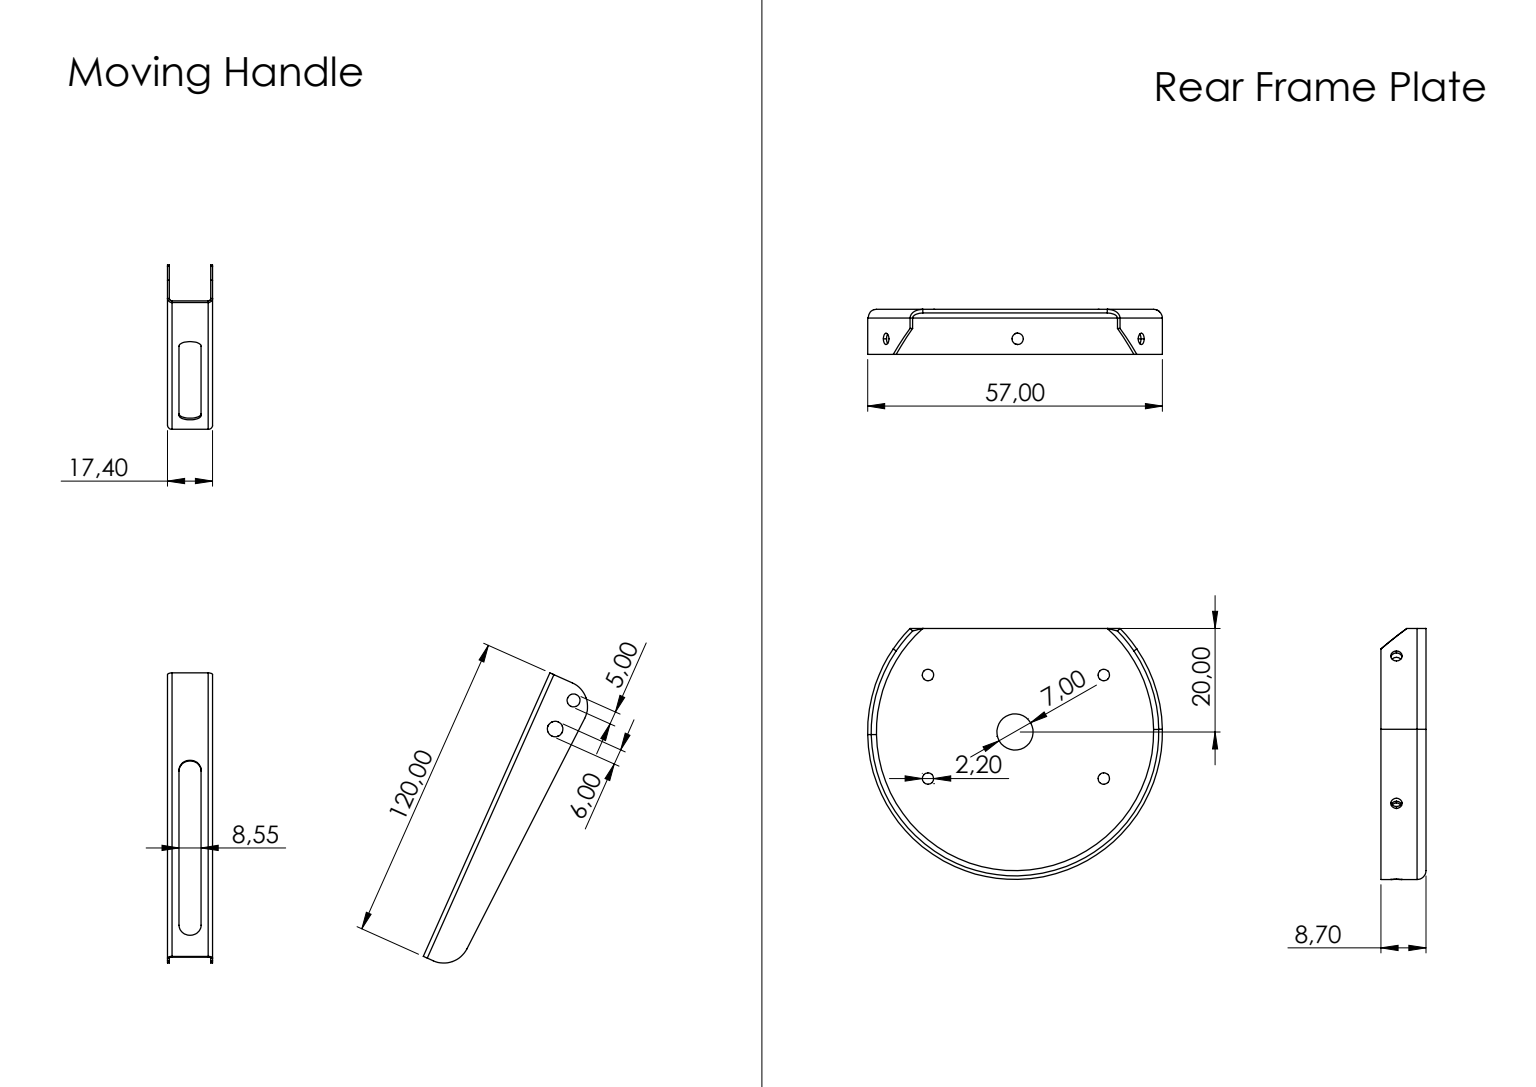
ISO-10303-21;
HEADER;
FILE_DESCRIPTION (('STEP AP214'),
    '1' );
FILE_NAME ('Moving Handle.step',
    '2026-10-06T09:00:30',
    ( '' ),
    ( '' ),
    'SwSTEP 2.0',
    'SolidWorks 2020',
    '' );
FILE_SCHEMA (( 'AUTOMOTIVE_DESIGN' ));
ENDSEC;

DATA;
#1=CARTESIAN_POINT ( 'NONE',  ( 7.707106781468556100, -5.692566302608600637, -27.29492475672613594 ) ) ;
#2=DIRECTION ( 'NONE',  ( 0.000000000000000000, 0.9128796883888953273, -0.4082287037029530552 ) ) ;
#16=VERTEX_POINT ( 'NONE', #10421 ) ;
#17=PRODUCT_DEFINITION ( 'UNKNOWN', '', #18877, #12195 ) ;
#34=DIRECTION ( 'NONE',  ( 1.000000000000000000, 3.839471067133294241E-11, -1.287095525146219562E-11 ) ) ;
#52=CARTESIAN_POINT ( 'NONE',  ( 1.057488903014505443E-10, -106.9648224075757952, 18.31364292107395642 ) ) ;
#61=VERTEX_POINT ( 'NONE', #24738 ) ;
#62=CARTESIAN_POINT ( 'NONE',  ( 7.707106781302665688, -60.46534760594231983, -2.801202534548945966 ) ) ;
#90=VERTEX_POINT ( 'NONE', #28021 ) ;
#95=DIRECTION ( 'NONE',  ( 2.764840495839172918E-12, 0.9128796883888953273, -0.4082287037029530552 ) ) ;
#99=CARTESIAN_POINT ( 'NONE',  ( 7.000000000111516130, -60.34578018690756807, -2.533826264242911908 ) ) ;
#105=DIRECTION ( 'NONE',  ( -1.000000000000000000, 5.687697937797165957E-16, -6.771501495045624776E-12 ) ) ;
#107=EDGE_CURVE ( 'NONE', #7680, #17625, #27535, .T. ) ;
#124=CARTESIAN_POINT ( 'NONE',  ( 7.291979204365766520, -115.1332600680515981, 21.92702704693240179 ) ) ;
#136=CARTESIAN_POINT ( 'NONE',  ( -7.000000000050451199, -115.5267901941139144, 21.04701626956108029 ) ) ;
#173=ORIENTED_EDGE ( 'NONE', *, *, #3047, .T. ) ;
#188=LINE ( 'NONE', #19684, #28372 ) ;
#203=ORIENTED_EDGE ( 'NONE', *, *, #5628, .T. ) ;
#223=DIRECTION ( 'NONE',  ( 1.000000000000000000, -1.843431230200084908E-12, 2.650498504963248473E-12 ) ) ;
#227=DIRECTION ( 'NONE',  ( 1.000000000000000000, -1.843431230200084908E-12, 2.650498504963248473E-12 ) ) ;
#233=LINE ( 'NONE', #19574, #18492 ) ;
#236=CARTESIAN_POINT ( 'NONE',  ( -8.000000000474178918, -29.73863906514523947, -27.17531388891475075 ) ) ;
#256=DIRECTION ( 'NONE',  ( -2.764840495839172918E-12, -0.9128796883888953273, 0.4082287037029531107 ) ) ;
#259=CARTESIAN_POINT ( 'NONE',  ( 8.000000000495651520, -23.99023929168359714, -28.09088344023833983 ) ) ;
#268=CARTESIAN_POINT ( 'NONE',  ( 8.700000000289421109, -16.34566964816854195, -38.02266470773063389 ) ) ;
#273=CARTESIAN_POINT ( 'NONE',  ( -8.699999999730765765, -25.41515418226572365, -25.82241997913822473 ) ) ;
#299=ORIENTED_EDGE ( 'NONE', *, *, #13486, .T. ) ;
#331=B_SPLINE_CURVE_WITH_KNOTS ( 'NONE', 4,
 ( #20135, #6279, #8153, #24861, #17748 ),
 .UNSPECIFIED., .F., .F.,
 ( 5, 5 ),
 ( -0.9817477042469999748, 0.9817477042469999748 ),
 .UNSPECIFIED. ) ;
#337=DIRECTION ( 'NONE',  ( -1.000000000000000000, 5.687697913155423197E-16, -6.771501495041734442E-12 ) ) ;
#360=LINE ( 'NONE', #2855, #2718 ) ;
#368=VERTEX_POINT ( 'NONE', #1564 ) ;
#371=ADVANCED_FACE ( 'NONE', ( #30354 ), #16338, .F. ) ;
#383=LINE ( 'NONE', #6989, #23905 ) ;
#402=EDGE_CURVE ( 'NONE', #3946, #1905, #1953, .T. ) ;
#419=CARTESIAN_POINT ( 'NONE',  ( 8.700000000293144353, -9.427296937348389250, -35.64651715365807405 ) ) ;
#421=EDGE_CURVE ( 'NONE', #12111, #14873, #20589, .T. ) ;
#435=LINE ( 'NONE', #22127, #18791 ) ;
#436=CARTESIAN_POINT ( 'NONE',  ( -7.999999999681902452, -14.92844969907143771, -33.25053330396754347 ) ) ;
#438=MANIFOLD_SOLID_BREP ( 'Stock-MAS-156-1', #10548 ) ;
#440=CARTESIAN_POINT ( 'NONE',  ( 7.665314379936610578, -115.2210683807244038, 21.73067038611315382 ) ) ;
#445=DIRECTION ( 'NONE',  ( -3.924189347185962345E-12, 0.4082287037029531107, 0.9128796883888953273 ) ) ;
#450=AXIS2_PLACEMENT_3D ( 'NONE', #30643, #26222, #11742 ) ;
#464=DIRECTION ( 'NONE',  ( -1.667070188605962886E-12, 0.4082287037029531107, 0.9128796883888953273 ) ) ;
#465=VECTOR ( 'NONE', #12974, 1000.000000000000000 ) ;
#469=DIRECTION ( 'NONE',  ( 2.764840495839172918E-12, 0.9128796883888953273, -0.4082287037029531107 ) ) ;
#475=CARTESIAN_POINT ( 'NONE',  ( 8.699999999949442397, -116.5561065468441626, 18.74526241745003574 ) ) ;
#492=DIRECTION ( 'NONE',  ( 6.325958275728752229E-12, 0.3568421334038983650, -0.9341647027306021478 ) ) ;
#496=EDGE_CURVE ( 'NONE', #28185, #6097, #18826, .T. ) ;
#531=CARTESIAN_POINT ( 'NONE',  ( -7.999999999670753148, -18.01685129643773564, -34.09892490238275542 ) ) ;
#545=CARTESIAN_POINT ( 'NONE',  ( -8.699999999716542476, -29.98791884354844939, -27.92359244214648228 ) ) ;
#555=CARTESIAN_POINT ( 'NONE',  ( -8.699999999672870743, -17.90468864316765973, -33.94136269864641520 ) ) ;
#575=CARTESIAN_POINT ( 'NONE',  ( -7.999999999684056284, -16.63651352361650382, -33.12749869627004529 ) ) ;
#597=ORIENTED_EDGE ( 'NONE', *, *, #20203, .T. ) ;
#605=VECTOR ( 'NONE', #18518, 1000.000000000000000 ) ;
#611=EDGE_LOOP ( 'NONE', ( #22896, #7545, #4645, #11032, #905, #16835, #7239, #10300 ) ) ;
#615=ADVANCED_FACE ( 'NONE', ( #10188, #8422, #29835 ), #7814, .F. ) ;
#617=CARTESIAN_POINT ( 'NONE',  ( 8.349999999579441834, -116.5561065468438215, 18.74526241744838373 ) ) ;
#624=CARTESIAN_POINT ( 'NONE',  ( -7.999999999945726081, -112.1477080532550445, 5.846459785100098117 ) ) ;
#657=CARTESIAN_POINT ( 'NONE',  ( 8.000000000883357387, -67.40749995174687115, -17.04319545456667484 ) ) ;
#713=EDGE_CURVE ( 'NONE', #20972, #5752, #15843, .T. ) ;
#714=CARTESIAN_POINT ( 'NONE',  ( -8.000000000001699973, -117.5009442568067755, 14.55791348096084192 ) ) ;
#725=VERTEX_POINT ( 'NONE', #10962 ) ;
#730=CARTESIAN_POINT ( 'NONE',  ( 7.000000000276031642, -5.430118837459354530, -26.70804059584096635 ) ) ;
#739=CARTESIAN_POINT ( 'NONE',  ( -7.999999999681398855, -14.76903124974032977, -33.32608274503188994 ) ) ;
#744=CYLINDRICAL_SURFACE ( 'NONE', #29818, 3.000000000000002220 ) ;
#754=CARTESIAN_POINT ( 'NONE',  ( -7.999999999888485647, -60.34578018689373380, -2.533826264313577603 ) ) ;
#757=CARTESIAN_POINT ( 'NONE',  ( 8.700000000279958456, -18.28438020625039329, -36.42481760783426381 ) ) ;
#773=CARTESIAN_POINT ( 'NONE',  ( -7.999999999947260854, -112.5823803020635125, 6.087179798330493163 ) ) ;
#775=DIRECTION ( 'NONE',  ( -1.000000000000000000, 5.687697999151106851E-16, -6.771501495036750356E-12 ) ) ;
#785=ORIENTED_EDGE ( 'NONE', *, *, #9500, .F. ) ;
#812=CARTESIAN_POINT ( 'NONE',  ( -8.699999999655181782, -13.66682223737418944, -36.55330428419230060 ) ) ;
#820=CARTESIAN_POINT ( 'NONE',  ( 7.785475348737113777, -115.2733928504967764, 21.61366257841296701 ) ) ;
#824=ORIENTED_EDGE ( 'NONE', *, *, #27429, .T. ) ;
#829=DIRECTION ( 'NONE',  ( 6.181308505765962611E-12, -0.4082287037029531107, -0.9128796883888953273 ) ) ;
#831=ORIENTED_EDGE ( 'NONE', *, *, #20654, .T. ) ;
#835=CARTESIAN_POINT ( 'NONE',  ( -7.999999999655180716, -13.66682223735657864, -36.55330428419717492 ) ) ;
#857=ORIENTED_EDGE ( 'NONE', *, *, #6995, .T. ) ;
#896=B_SPLINE_CURVE_WITH_KNOTS ( 'NONE', 3,
 ( #3635, #22846, #20952, #8825, #16225, #8506 ),
 .UNSPECIFIED., .F., .F.,
 ( 4, 2, 4 ),
 ( 0.000000000000000000, 0.5000000000000000000, 1.000000000000000000 ),
 .UNSPECIFIED. ) ;
#905=ORIENTED_EDGE ( 'NONE', *, *, #2120, .T. ) ;
#912=CARTESIAN_POINT ( 'NONE',  ( 8.700000000283074186, -17.54022835462044227, -37.48857263400110895 ) ) ;
#914=CYLINDRICAL_SURFACE ( 'NONE', #15454, 3.000000000000002220 ) ;
#945=CARTESIAN_POINT ( 'NONE',  ( 8.000000000289732682, -15.05691661385925961, -37.86814300156539304 ) ) ;
#950=DIRECTION ( 'NONE',  ( 3.924189347185962345E-12, -0.4082287037029530552, -0.9128796883888953273 ) ) ;
#954=DIRECTION ( 'NONE',  ( -1.000000000000000000, 5.687697999151106851E-16, -6.771501495036750356E-12 ) ) ;
#972=CARTESIAN_POINT ( 'NONE',  ( -7.999999999697742226, -24.65319937755806379, -30.30964379067835424 ) ) ;
#983=CARTESIAN_POINT ( 'NONE',  ( -7.999999999652784410, -17.12901166691730737, -37.73938230484767331 ) ) ;
#989=CARTESIAN_POINT ( 'NONE',  ( -7.999999999658122363, -13.45788390610263541, -35.88763790175109136 ) ) ;
#1016=EDGE_CURVE ( 'NONE', #725, #3834, #25246, .T. ) ;
#1017=CARTESIAN_POINT ( 'NONE',  ( -8.699999999945166707, -111.9817663798742444, 5.760339591697572814 ) ) ;
#1020=EDGE_CURVE ( 'NONE', #9868, #26249, #30013, .T. ) ;
#1081=DIRECTION ( 'NONE',  ( -1.000000000000000000, 5.687697999151106851E-16, -6.771501495036750356E-12 ) ) ;
#1113=EDGE_CURVE ( 'NONE', #7730, #30387, #4258, .T. ) ;
#1116=EDGE_LOOP ( 'NONE', ( #4416, #12493, #12956, #27444 ) ) ;
#1192=DIRECTION ( 'NONE',  ( 1.000000000000000000, -9.219999999999999084E-13, 4.710999999999999616E-12 ) ) ;
#1197=B_SPLINE_CURVE_WITH_KNOTS ( 'NONE', 3,
 ( #19881, #13084, #10731, #4703, #11053, #9258 ),
 .UNSPECIFIED., .F., .F.,
 ( 4, 2, 4 ),
 ( 0.000000000000000000, 0.5000000000000000000, 1.000000000000000000 ),
 .UNSPECIFIED. ) ;
#1198=EDGE_CURVE ( 'NONE', #2707, #23086, #13529, .T. ) ;
#1223=DIRECTION ( 'NONE',  ( 1.520059509754405802E-12, -0.4554456718803465698, -0.8902635789278700029 ) ) ;
#1253=FACE_OUTER_BOUND ( 'NONE', #18893, .T. ) ;
#1280=ORIENTED_EDGE ( 'NONE', *, *, #3659, .F. ) ;
#1289=DIRECTION ( 'NONE',  ( 1.000000000000000000, -1.843431230200084908E-12, 2.650498504963248473E-12 ) ) ;
#1311=DIRECTION ( 'NONE',  ( -1.000000000000000000, 5.687698019341907056E-16, -6.771501495046482653E-12 ) ) ;
#1331=CARTESIAN_POINT ( 'NONE',  ( 8.699999999994835420, -111.9817663798902885, 5.760339591779549018 ) ) ;
#1361=ORIENTED_EDGE ( 'NONE', *, *, #16817, .F. ) ;
#1401=ORIENTED_EDGE ( 'NONE', *, *, #2120, .F. ) ;
#1404=ADVANCED_FACE ( 'NONE', ( #13306 ), #27776, .F. ) ;
#1432=EDGE_LOOP ( 'NONE', ( #299, #9426, #4454, #14051 ) ) ;
#1440=CIRCLE ( 'NONE', #9974, 10.00000000000000355 ) ;
#1443=EDGE_CURVE ( 'NONE', #12111, #5252, #1887, .T. ) ;
#1446=CARTESIAN_POINT ( 'NONE',  ( -8.699999998997657968, -25.77531388886905006, -25.66136093486021608 ) ) ;
#1456=EDGE_LOOP ( 'NONE', ( #28511, #8580, #30468, #16902, #27099, #12265, #27129, #24342 ) ) ;
#1477=AXIS2_PLACEMENT_3D ( 'NONE', #30131, #20218, #29810 ) ;
#1480=DIRECTION ( 'NONE',  ( 3.134067079931429195E-12, 0.3568421334038983650, -0.9341647027306021478 ) ) ;
#1481=ORIENTED_EDGE ( 'NONE', *, *, #24442, .T. ) ;
#1509=CYLINDRICAL_SURFACE ( 'NONE', #21807, 2.500000000000000888 ) ;
#1512=DIRECTION ( 'NONE',  ( -3.924189347185963153E-12, 0.4082287037029530552, 0.9128796883888953273 ) ) ;
#1530=CARTESIAN_POINT ( 'NONE',  ( 8.000000000281330514, -5.981227587277713198, -27.94042817480428198 ) ) ;
#1538=CARTESIAN_POINT ( 'NONE',  ( -8.699999999715409160, -23.99014701217026513, -28.09041065100222312 ) ) ;
#1539=DIRECTION ( 'NONE',  ( -1.000000000000000000, 5.687697913153403713E-16, -6.771501495041734442E-12 ) ) ;
#1541=CARTESIAN_POINT ( 'NONE',  ( -7.999999999712662735, -24.01208138055985941, -28.87597782795289802 ) ) ;
#1542=PLANE ( 'NONE',  #10003 ) ;
#1546=CARTESIAN_POINT ( 'NONE',  ( 7.999999999977091214, -107.4273096626279482, 14.66297538114749344 ) ) ;
#1561=ORIENTED_EDGE ( 'NONE', *, *, #20981, .T. ) ;
#1562=EDGE_LOOP ( 'NONE', ( #10993, #30576, #17167, #18297 ) ) ;
#1564=CARTESIAN_POINT ( 'NONE',  ( -8.699999999681903518, -14.92844969908904851, -33.25053330396269047 ) ) ;
#1570=CARTESIAN_POINT ( 'NONE',  ( 8.000000000232340369, -25.77531388888444752, -25.66136093478154123 ) ) ;
#1575=ADVANCED_FACE ( 'NONE', ( #17176 ), #5217, .T. ) ;
#1599=CARTESIAN_POINT ( 'NONE',  ( -6.999999999262594308, -5.572998883415898774, -27.02754848611273530 ) ) ;
#1602=CARTESIAN_POINT ( 'NONE',  ( 8.000000000836740455, -15.37655846826601014, -33.05014450755139421 ) ) ;
#1617=LINE ( 'NONE', #20810, #27270 ) ;
#1628=ORIENTED_EDGE ( 'NONE', *, *, #2753, .F. ) ;
#1638=CARTESIAN_POINT ( 'NONE',  ( 8.699999999564820286, -13.66682223739023350, -36.55330428411032528 ) ) ;
#1646=CARTESIAN_POINT ( 'NONE',  ( 8.699999999979134202, -115.7892272573602668, 9.034522711534439310 ) ) ;
#1650=DIRECTION ( 'NONE',  ( -1.000000000000000000, 5.687697993419811493E-16, -6.771501495049272772E-12 ) ) ;
#1653=ORIENTED_EDGE ( 'NONE', *, *, #4274, .T. ) ;
#1675=ORIENTED_EDGE ( 'NONE', *, *, #19444, .T. ) ;
#1701=FACE_OUTER_BOUND ( 'NONE', #27105, .T. ) ;
#1705=ORIENTED_EDGE ( 'NONE', *, *, #20203, .F. ) ;
#1724=ORIENTED_EDGE ( 'NONE', *, *, #1020, .T. ) ;
#1729=B_SPLINE_CURVE_WITH_KNOTS ( 'NONE', 3,
 ( #3155, #17170, #5061, #26934, #19388, #7722 ),
 .UNSPECIFIED., .F., .F.,
 ( 4, 2, 4 ),
 ( 0.000000000000000000, 0.5000000000000000000, 1.000000000000000000 ),
 .UNSPECIFIED. ) ;
#1738=CARTESIAN_POINT ( 'NONE',  ( 7.614137047270383540, -5.654631194664418992, -27.21009439270542885 ) ) ;
#1748=VERTEX_POINT ( 'NONE', #6457 ) ;
#1754=ORIENTED_EDGE ( 'NONE', *, *, #30180, .F. ) ;
#1768=ORIENTED_EDGE ( 'NONE', *, *, #496, .F. ) ;
#1772=AXIS2_PLACEMENT_3D ( 'NONE', #11123, #11436, #18818 ) ;
#1787=DIRECTION ( 'NONE',  ( 1.000000000000000000, -9.219999999999999084E-13, 4.710999999999999616E-12 ) ) ;
#1789=ORIENTED_EDGE ( 'NONE', *, *, #16604, .F. ) ;
#1828=VERTEX_POINT ( 'NONE', #24929 ) ;
#1834=ORIENTED_EDGE ( 'NONE', *, *, #16604, .T. ) ;
#1842=CYLINDRICAL_SURFACE ( 'NONE', #13013, 2.500000000000002220 ) ;
#1869=CARTESIAN_POINT ( 'NONE',  ( 8.700000000277906764, -15.94902145836247342, -35.53273252485295330 ) ) ;
#1887=B_SPLINE_CURVE_WITH_KNOTS ( 'NONE', 3,
 ( #23076, #22606, #13141, #11110, #18341, #27943 ),
 .UNSPECIFIED., .F., .F.,
 ( 4, 2, 4 ),
 ( 0.000000000000000000, 0.5000000000000000000, 1.000000000000000000 ),
 .UNSPECIFIED. ) ;
#1891=CARTESIAN_POINT ( 'NONE',  ( 8.700000000233908182, -29.89969810940666406, -27.53547359536790395 ) ) ;
#1899=DIRECTION ( 'NONE',  ( -1.000000000000000000, 5.687697999151106851E-16, -6.771501495036750356E-12 ) ) ;
#1900=ORIENTED_EDGE ( 'NONE', *, *, #25212, .T. ) ;
#1903=EDGE_CURVE ( 'NONE', #19512, #21002, #23668, .T. ) ;
#1905=VERTEX_POINT ( 'NONE', #1017 ) ;
#1925=VECTOR ( 'NONE', #13869, 1000.000000000000000 ) ;
#1943=ORIENTED_EDGE ( 'NONE', *, *, #7815, .T. ) ;
#1953=B_SPLINE_CURVE_WITH_KNOTS ( 'NONE', 3,
 ( #25642, #6882, #11469, #4071, #21215, #11154 ),
 .UNSPECIFIED., .F., .F.,
 ( 4, 2, 4 ),
 ( 0.000000000000000000, 0.5000000000000001110, 1.000000000000000000 ),
 .UNSPECIFIED. ) ;
#1968=CARTESIAN_POINT ( 'NONE',  ( 8.000000000363138852, -29.66236253008535328, -29.83737202107615971 ) ) ;
#1978=ORIENTED_EDGE ( 'NONE', *, *, #2333, .F. ) ;
#2016=CARTESIAN_POINT ( 'NONE',  ( 8.700000000286559398, -7.565603753668719733, -31.48340496194444782 ) ) ;
#2049=CARTESIAN_POINT ( 'NONE',  ( -8.699999999715885224, -26.99999999997790923, -28.40000000002690683 ) ) ;
#2050=CYLINDRICAL_SURFACE ( 'NONE', #20849, 10.00000000000000178 ) ;
#2058=VERTEX_POINT ( 'NONE', #13425 ) ;
#2081=DIRECTION ( 'NONE',  ( 1.000000000000000000, -9.219999999999999084E-13, 4.710999999999999616E-12 ) ) ;
#2102=CARTESIAN_POINT ( 'NONE',  ( -8.699999999651183202, -14.46922738198402136, -37.57413277573995458 ) ) ;
#2105=AXIS2_PLACEMENT_3D ( 'NONE', #20895, #1223, #18035 ) ;
#2109=VECTOR ( 'NONE', #2270, 1000.000000000000114 ) ;
#2114=DIRECTION ( 'NONE',  ( 6.386904893851405129E-12, 0.3322662713817149949, -0.9431856258987901809 ) ) ;
#2120=EDGE_CURVE ( 'NONE', #17525, #17033, #24050, .T. ) ;
#2124=DIRECTION ( 'NONE',  ( 1.000000000000000000, -9.219999999999999084E-13, 4.710999999999999616E-12 ) ) ;
#2127=CARTESIAN_POINT ( 'NONE',  ( -7.999999999667107176, -18.39629690576770926, -34.94743992953217315 ) ) ;
#2150=UNCERTAINTY_MEASURE_WITH_UNIT (LENGTH_MEASURE( 1.000000000000000082E-05 ), #3991, 'distance_accuracy_value', 'NONE');
#2151=FACE_OUTER_BOUND ( 'NONE', #4462, .T. ) ;
#2152=EDGE_CURVE ( 'NONE', #27598, #22033, #3753, .T. ) ;
#2171=ORIENTED_EDGE ( 'NONE', *, *, #30137, .F. ) ;
#2178=B_SPLINE_CURVE_WITH_KNOTS ( 'NONE', 3,
 ( #4961, #2456, #259, #26825, #12502, #17072 ),
 .UNSPECIFIED., .F., .F.,
 ( 4, 2, 4 ),
 ( 0.000000000000000000, 0.5000000000000000000, 1.000000000000000000 ),
 .UNSPECIFIED. ) ;
#2182=AXIS2_PLACEMENT_3D ( 'NONE', #9189, #6836, #18789 ) ;
#2183=CARTESIAN_POINT ( 'NONE',  ( -8.699999999652812122, -10.55555246029782346, -37.33318641903195356 ) ) ;
#2184=CYLINDRICAL_SURFACE ( 'NONE', #12936, 2.500000000000000888 ) ;
#2214=CARTESIAN_POINT ( 'NONE',  ( -7.999999999655180716, -13.66682223735657864, -36.55330428419717492 ) ) ;
#2250=DIRECTION ( 'NONE',  ( 0.000000000000000000, -0.9128796883888953273, 0.4082287037029526666 ) ) ;
#2253=FACE_OUTER_BOUND ( 'NONE', #30967, .T. ) ;
#2259=ORIENTED_EDGE ( 'NONE', *, *, #7317, .T. ) ;
#2270=DIRECTION ( 'NONE',  ( -3.924189347185961537E-12, 0.4082287037029530552, 0.9128796883888952163 ) ) ;
#2280=B_SPLINE_CURVE_WITH_KNOTS ( 'NONE', 3,
 ( #9784, #15895, #15421, #20453, #18079, #8024 ),
 .UNSPECIFIED., .F., .F.,
 ( 4, 2, 4 ),
 ( 0.000000000000000000, 0.5000000000000000000, 1.000000000000000000 ),
 .UNSPECIFIED. ) ;
#2306=EDGE_LOOP ( 'NONE', ( #11495, #9641, #26655, #18802 ) ) ;
#2310=CARTESIAN_POINT ( 'NONE',  ( 8.700000000294076941, -9.763850040216345505, -36.23184806385972934 ) ) ;
#2333=EDGE_CURVE ( 'NONE', #23754, #8842, #22384, .T. ) ;
#2336=ORIENTED_EDGE ( 'NONE', *, *, #2412, .T. ) ;
#2357=CARTESIAN_POINT ( 'NONE',  ( 8.700000000235821318, -29.73863906516063693, -27.17531388883607590 ) ) ;
#2399=DIRECTION ( 'NONE',  ( -1.000000000000000000, 5.687697999151106851E-16, -6.771501495036750356E-12 ) ) ;
#2404=DIRECTION ( 'NONE',  ( 3.924189347185962345E-12, -0.4082287037029530552, -0.9128796883888953273 ) ) ;
#2412=EDGE_CURVE ( 'NONE', #16, #8184, #25150, .T. ) ;
#2420=FACE_OUTER_BOUND ( 'NONE', #9603, .T. ) ;
#2430=DIRECTION ( 'NONE',  ( -1.000000000000000000, 5.687697999151106851E-16, -6.771501495036750356E-12 ) ) ;
#2432=B_SPLINE_CURVE_WITH_KNOTS ( 'NONE', 3,
 ( #19714, #2564, #21611, #14683, #5225, #7127 ),
 .UNSPECIFIED., .F., .F.,
 ( 4, 2, 4 ),
 ( 0.000000000000000000, 0.5000000000000000000, 1.000000000000000000 ),
 .UNSPECIFIED. ) ;
#2445=ORIENTED_EDGE ( 'NONE', *, *, #24054, .T. ) ;
#2456=CARTESIAN_POINT ( 'NONE',  ( 8.000000000368686415, -24.05737431370143398, -27.69631922065391905 ) ) ;
#2459=CARTESIAN_POINT ( 'NONE',  ( 8.700000000285857737, -13.61366271048277277, -34.64064744186795508 ) ) ;
#2499=VERTEX_POINT ( 'NONE', #30665 ) ;
#2515=B_SPLINE_CURVE_WITH_KNOTS ( 'NONE', 3,
 ( #4871, #10058, #7677, #23925, #12407, #475 ),
 .UNSPECIFIED., .F., .F.,
 ( 4, 2, 4 ),
 ( 0.000000000000000000, 0.5000000000000000000, 1.000000000000000000 ),
 .UNSPECIFIED. ) ;
#2529=FACE_OUTER_BOUND ( 'NONE', #4143, .T. ) ;
#2532=CARTESIAN_POINT ( 'NONE',  ( -8.699999999662093586, -15.94902145834643115, -35.53273252493492862 ) ) ;
#2542=DIRECTION ( 'NONE',  ( 1.000000000000000000, -1.843431230200084908E-12, 2.650498504963248473E-12 ) ) ;
#2564=CARTESIAN_POINT ( 'NONE',  ( -7.799123028745747810, -5.730129976181659757, -27.37892452043196556 ) ) ;
#2567=CARTESIAN_POINT ( 'NONE',  ( -4.276011752185619130, -110.9401521130015027, -1.050525799534463012 ) ) ;
#2576=B_SPLINE_CURVE_WITH_KNOTS ( 'NONE', 3,
 ( #4173, #18790, #11253, #21474, #16438, #9190 ),
 .UNSPECIFIED., .F., .F.,
 ( 4, 2, 4 ),
 ( 0.000000000000000000, 0.5000000000000000000, 1.000000000000000000 ),
 .UNSPECIFIED. ) ;
#2605=CARTESIAN_POINT ( 'NONE',  ( -7.999999999682589014, -15.17486759261230311, -33.15315993661145910 ) ) ;
#2609=CARTESIAN_POINT ( 'NONE',  ( 8.700000000287717583, -16.96959321760160222, -37.81493174583334849 ) ) ;
#2615=CARTESIAN_POINT ( 'NONE',  ( -8.699999999718343702, -24.19750589173278499, -27.32947359979484858 ) ) ;
#2619=EDGE_CURVE ( 'NONE', #16921, #22622, #17600, .T. ) ;
#2627=CARTESIAN_POINT ( 'NONE',  ( 0.000000000000000000, 0.000000000000000000, 0.000000000000000000 ) ) ;
#2638=( NAMED_UNIT ( * ) SI_UNIT ( $, .STERADIAN. ) SOLID_ANGLE_UNIT ( ) );
#2641=DIRECTION ( 'NONE',  ( -1.000000000000000000, 5.687698019341907056E-16, -6.771501495046482653E-12 ) ) ;
#2651=VECTOR ( 'NONE', #7343, 1000.000000000000114 ) ;
#2669=ORIENTED_EDGE ( 'NONE', *, *, #30970, .T. ) ;
#2673=CARTESIAN_POINT ( 'NONE',  ( -7.999999999729513256, -26.54727805893419657, -25.41789611383235226 ) ) ;
#2689=EDGE_CURVE ( 'NONE', #18386, #18002, #22877, .T. ) ;
#2707=VERTEX_POINT ( 'NONE', #11920 ) ;
#2717=CARTESIAN_POINT ( 'NONE',  ( -7.999999999683915952, -16.84112630284391443, -33.19732204833458411 ) ) ;
#2718=VECTOR ( 'NONE', #4910, 1000.000000000000000 ) ;
#2753=EDGE_CURVE ( 'NONE', #15244, #5752, #12004, .T. ) ;
#2756=VERTEX_POINT ( 'NONE', #10496 ) ;
#2770=CYLINDRICAL_SURFACE ( 'NONE', #28345, 3.000000000000002220 ) ;
#2785=VERTEX_POINT ( 'NONE', #21181 ) ;
#2801=CARTESIAN_POINT ( 'NONE',  ( 8.700000000244115128, -26.99999999999395328, -28.39999999994493862 ) ) ;
#2821=ORIENTED_EDGE ( 'NONE', *, *, #9836, .F. ) ;
#2855=CARTESIAN_POINT ( 'NONE',  ( 8.699999999511655702, -24.19750589174882904, -27.32947359971288037 ) ) ;
#2866=CARTESIAN_POINT ( 'NONE',  ( 8.700000000252410715, -24.26136093482726608, -29.62468611105379779 ) ) ;
#2868=DIRECTION ( 'NONE',  ( -3.924189347185962345E-12, 0.4082287037029531107, 0.9128796883888953273 ) ) ;
#2879=LINE ( 'NONE', #28840, #12838 ) ;
#2908=EDGE_CURVE ( 'NONE', #13888, #17663, #7099, .T. ) ;
#2913=EDGE_CURVE ( 'NONE', #23040, #9577, #12648, .T. ) ;
#2914=CARTESIAN_POINT ( 'NONE',  ( -7.999999999668208517, -9.149979920084513552, -35.02638174925785819 ) ) ;
#2924=AXIS2_PLACEMENT_3D ( 'NONE', #17301, #337, #492 ) ;
#2957=VECTOR ( 'NONE', #27758, 999.9999999999998863 ) ;
#2967=ADVANCED_FACE ( 'NONE', ( #20992 ), #9023, .F. ) ;
#2969=LINE ( 'NONE', #15231, #26882 ) ;
#2989=CARTESIAN_POINT ( 'NONE',  ( 5.797918472256613498, -5.490503403373238278, -26.84307236410781172 ) ) ;
#2998=CARTESIAN_POINT ( 'NONE',  ( -6.999999999884560786, -60.75400889059761766, -3.446705952697758590 ) ) ;
#3021=CARTESIAN_POINT ( 'NONE',  ( -7.999999999659364924, -18.23057825131764531, -36.55854538514943641 ) ) ;
#3022=ORIENTED_EDGE ( 'NONE', *, *, #2152, .T. ) ;
#3036=CARTESIAN_POINT ( 'NONE',  ( -8.699999999786642846, -67.40749995144571471, -17.04319545400634084 ) ) ;
#3043=FACE_OUTER_BOUND ( 'NONE', #28369, .T. ) ;
#3047=EDGE_CURVE ( 'NONE', #3834, #17179, #12007, .T. ) ;
#3055=DIRECTION ( 'NONE',  ( 0.000000000000000000, -0.9128796883888952163, 0.4082287037029533328 ) ) ;
#3113=CYLINDRICAL_SURFACE ( 'NONE', #30869, 2.500000000000001776 ) ;
#3128=APPLICATION_CONTEXT ( 'automotive_design' ) ;
#3134=LINE ( 'NONE', #19975, #24510 ) ;
#3137=LINE ( 'NONE', #12736, #9564 ) ;
#3152=CARTESIAN_POINT ( 'NONE',  ( -8.699999999674142614, -13.61360970150653316, -34.64062719139432289 ) ) ;
#3155=CARTESIAN_POINT ( 'NONE',  ( 8.000000000232340369, -25.77531388888444752, -25.66136093478154123 ) ) ;
#3194=CARTESIAN_POINT ( 'NONE',  ( -8.699999999677118012, -17.14683147485207471, -33.31409708255895907 ) ) ;
#3207=CARTESIAN_POINT ( 'NONE',  ( -8.000000000018781421, -117.3918542544958115, 16.08262865818876008 ) ) ;
#3253=LINE ( 'NONE', #29532, #5771 ) ;
#3259=DIRECTION ( 'NONE',  ( -1.000000000000000000, 5.687698019341907056E-16, -6.771501495046482653E-12 ) ) ;
#3284=ADVANCED_FACE ( 'NONE', ( #12463 ), #24900, .F. ) ;
#3323=CARTESIAN_POINT ( 'NONE',  ( -7.999999999655324601, -17.72367216628370556, -37.31664291223312091 ) ) ;
#3337=B_SPLINE_CURVE_WITH_KNOTS ( 'NONE', 3,
 ( #14013, #16823, #11646, #26274, #23618, #4410 ),
 .UNSPECIFIED., .F., .F.,
 ( 4, 2, 4 ),
 ( 0.000000000000000000, 0.5000000000000000000, 1.000000000000000000 ),
 .UNSPECIFIED. ) ;
#3356=CARTESIAN_POINT ( 'NONE',  ( -7.999999999988746779, -117.0548398251480364, 11.89578701954164686 ) ) ;
#3369=ORIENTED_EDGE ( 'NONE', *, *, #14073, .T. ) ;
#3390=DIRECTION ( 'NONE',  ( 2.764840495839172918E-12, 0.9128796883888953273, -0.4082287037029531107 ) ) ;
#3399=EDGE_CURVE ( 'NONE', #29694, #1748, #3493, .T. ) ;
#3428=ADVANCED_FACE ( 'NONE', ( #21893 ), #21580, .F. ) ;
#3461=CARTESIAN_POINT ( 'NONE',  ( -7.999999999728557576, -25.41682687375232064, -25.82167197182654661 ) ) ;
#3471=AXIS2_PLACEMENT_3D ( 'NONE', #22262, #26521, #24015 ) ;
#3484=ORIENTED_EDGE ( 'NONE', *, *, #21630, .T. ) ;
#3493=B_SPLINE_CURVE_WITH_KNOTS ( 'NONE', 3,
 ( #6468, #14181, #18736, #17000, #14346, #12276 ),
 .UNSPECIFIED., .F., .F.,
 ( 4, 2, 4 ),
 ( 0.000000000000000000, 0.5000000000000000000, 1.000000000000000000 ),
 .UNSPECIFIED. ) ;
#3494=VECTOR ( 'NONE', #22040, 1000.000000000000114 ) ;
#3501=FACE_OUTER_BOUND ( 'NONE', #30433, .T. ) ;
#3528=CARTESIAN_POINT ( 'NONE',  ( 7.000000000108768994, -60.06002009431549737, -1.894810482370685278 ) ) ;
#3550=B_SPLINE_CURVE_WITH_KNOTS ( 'NONE', 5,
 ( #29442, #22375, #22215, #820, #14831, #10410, #17480, #17778, #27391, #5830, #21918, #19549 ),
 .UNSPECIFIED., .F., .F.,
 ( 6, 3, 3, 6 ),
 ( 1.117931991990000151, 1.394586747660000015, 2.091870620439999939, 2.235835859519999858 ),
 .UNSPECIFIED. ) ;
#3556=CARTESIAN_POINT ( 'NONE',  ( 8.700000000294906499, -15.59658250094199161, -40.60120179151234510 ) ) ;
#3562=CARTESIAN_POINT ( 'NONE',  ( -8.699999999715885224, -26.99999999997790923, -28.40000000002690683 ) ) ;
#3585=ORIENTED_EDGE ( 'NONE', *, *, #14607, .F. ) ;
#3586=EDGE_CURVE ( 'NONE', #30810, #24995, #3137, .T. ) ;
#3600=ORIENTED_EDGE ( 'NONE', *, *, #18462, .F. ) ;
#3606=LINE ( 'NONE', #29737, #24715 ) ;
#3621=ORIENTED_EDGE ( 'NONE', *, *, #7436, .T. ) ;
#3623=VERTEX_POINT ( 'NONE', #1570 ) ;
#3634=PLANE ( 'NONE',  #23108 ) ;
#3635=CARTESIAN_POINT ( 'NONE',  ( -8.699999999642283655, -16.96959321760381556, -37.81493174590716677 ) ) ;
#3651=VERTEX_POINT ( 'NONE', #30193 ) ;
#3654=CARTESIAN_POINT ( 'NONE',  ( -8.699999999662093586, -15.94902145834643115, -35.53273252493492862 ) ) ;
#3659=EDGE_CURVE ( 'NONE', #15429, #30761, #24134, .T. ) ;
#3666=VERTEX_POINT ( 'NONE', #18221 ) ;
#3685=LINE ( 'NONE', #8391, #465 ) ;
#3711=ORIENTED_EDGE ( 'NONE', *, *, #10079, .T. ) ;
#3714=VECTOR ( 'NONE', #13963, 1000.000000000000000 ) ;
#3730=CARTESIAN_POINT ( 'NONE',  ( -7.999999999710018628, -24.10104989765104833, -29.26619909559191157 ) ) ;
#3753=B_SPLINE_CURVE_WITH_KNOTS ( 'NONE', 3,
 ( #19400, #5074, #2102, #28378, #9329, #9639 ),
 .UNSPECIFIED., .F., .F.,
 ( 4, 2, 4 ),
 ( 0.000000000000000000, 0.5000000000000000000, 1.000000000000000000 ),
 .UNSPECIFIED. ) ;
#3776=CARTESIAN_POINT ( 'NONE',  ( -7.999999999627967817, -15.63018644032419857, -40.59129444282516630 ) ) ;
#3801=DIRECTION ( 'NONE',  ( 1.000000000000000000, -1.843431230200084908E-12, 2.650498504963248473E-12 ) ) ;
#3834=VERTEX_POINT ( 'NONE', #21075 ) ;
#3850=ORIENTED_EDGE ( 'NONE', *, *, #27186, .F. ) ;
#3861=CARTESIAN_POINT ( 'NONE',  ( 6.999999999814658480, -5.287238791122498505, -26.38853270481357072 ) ) ;
#3869=DIRECTION ( 'NONE',  ( -2.415891560877031462E-12, 0.9341647027306021478, 0.3568421334038983650 ) ) ;
#3884=EDGE_CURVE ( 'NONE', #9121, #31008, #331, .T. ) ;
#3890=CARTESIAN_POINT ( 'NONE',  ( -8.699999999662093586, -15.94902145834643115, -35.53273252493492862 ) ) ;
#3906=VERTEX_POINT ( 'NONE', #25005 ) ;
#3908=ORIENTED_EDGE ( 'NONE', *, *, #13956, .T. ) ;
#3938=CYLINDRICAL_SURFACE ( 'NONE', #14271, 3.000000000000002220 ) ;
#3942=ORIENTED_EDGE ( 'NONE', *, *, #2689, .F. ) ;
#3946=VERTEX_POINT ( 'NONE', #30192 ) ;
#3956=CARTESIAN_POINT ( 'NONE',  ( 8.000000000465679051, -16.38256976572606405, -33.02215629541608877 ) ) ;
#3967=ADVANCED_FACE ( 'NONE', ( #1253 ), #18220, .T. ) ;
#3968=CARTESIAN_POINT ( 'NONE',  ( 7.999999999944494178, -116.0414483704652042, 19.89613934358488123 ) ) ;
#3991=( LENGTH_UNIT ( ) NAMED_UNIT ( * ) SI_UNIT ( .MILLI., .METRE. ) );
#4003=AXIS2_PLACEMENT_3D ( 'NONE', #754, #10646, #20238 ) ;
#4015=CARTESIAN_POINT ( 'NONE',  ( 8.000000000270995670, -18.23122067931581114, -34.51216076560703527 ) ) ;
#4042=FACE_OUTER_BOUND ( 'NONE', #18444, .T. ) ;
#4048=EDGE_CURVE ( 'NONE', #22923, #2058, #13991, .T. ) ;
#4060=CARTESIAN_POINT ( 'NONE',  ( -8.699999999642283655, -16.96959321760381556, -37.81493174590716677 ) ) ;
#4071=CARTESIAN_POINT ( 'NONE',  ( -8.699999999957434227, -114.1237136948164306, 7.129097339259313770 ) ) ;
#4073=CARTESIAN_POINT ( 'NONE',  ( -8.699999999664235872, -9.427153351153990002, -35.64619606679892883 ) ) ;
#4096=FACE_OUTER_BOUND ( 'NONE', #20301, .T. ) ;
#4136=EDGE_LOOP ( 'NONE', ( #10645, #7084, #21287, #19421 ) ) ;
#4138=DIRECTION ( 'NONE',  ( -3.927995826131583318E-12, 0.4082287037029531107, 0.9128796883888953273 ) ) ;
#4140=VECTOR ( 'NONE', #22590, 1000.000000000000000 ) ;
#4143=EDGE_LOOP ( 'NONE', ( #17592, #28862, #14441, #6769 ) ) ;
#4168=CARTESIAN_POINT ( 'NONE',  ( -8.699999999681903518, -14.92844969908904851, -33.25053330396269047 ) ) ;
#4173=CARTESIAN_POINT ( 'NONE',  ( 8.000000000245886866, -28.22468611110216230, -31.13863906511491209 ) ) ;
#4202=FACE_OUTER_BOUND ( 'NONE', #28460, .T. ) ;
#4212=CARTESIAN_POINT ( 'NONE',  ( 8.699999999974050269, -116.8589940799748632, 11.34037320843244956 ) ) ;
#4237=VERTEX_POINT ( 'NONE', #29840 ) ;
#4243=CARTESIAN_POINT ( 'NONE',  ( 8.000000000480120832, -27.30911655970313845, -25.39023929163792204 ) ) ;
#4244=CARTESIAN_POINT ( 'NONE',  ( -6.999999999718670374, -5.981227587263883372, -27.94042817487494901 ) ) ;
#4249=EDGE_CURVE ( 'NONE', #24850, #24204, #4401, .T. ) ;
#4258=LINE ( 'NONE', #27857, #13061 ) ;
#4274=EDGE_CURVE ( 'NONE', #22839, #9868, #3253, .T. ) ;
#4287=CYLINDRICAL_SURFACE ( 'NONE', #12133, 1.700000000000000178 ) ;
#4301=B_SPLINE_CURVE_WITH_KNOTS ( 'NONE', 3,
 ( #27035, #10514, #12707, #20113, #19953, #5472 ),
 .UNSPECIFIED., .F., .F.,
 ( 4, 2, 4 ),
 ( 0.000000000000000000, 0.5000000000000000000, 1.000000000000000000 ),
 .UNSPECIFIED. ) ;
#4306=ORIENTED_EDGE ( 'NONE', *, *, #7347, .F. ) ;
#4314=DIRECTION ( 'NONE',  ( 6.325958275728752229E-12, 0.3568421334038983650, -0.9341647027306021478 ) ) ;
#4320=CYLINDRICAL_SURFACE ( 'NONE', #21877, 10.00000000000000533 ) ;
#4328=ADVANCED_FACE ( 'NONE', ( #2151 ), #23091, .F. ) ;
#4333=DIRECTION ( 'NONE',  ( -3.924189347185963153E-12, 0.4082287037029530552, 0.9128796883888953273 ) ) ;
#4355=DIRECTION ( 'NONE',  ( -1.000000000000000000, 5.687697913153403713E-16, -6.771501495041734442E-12 ) ) ;
#4358=PLANE ( 'NONE',  #6731 ) ;
#4367=DIRECTION ( 'NONE',  ( -1.667070188605962886E-12, 0.4082287037029531107, 0.9128796883888953273 ) ) ;
#4378=PRODUCT_DEFINITION_SHAPE ( 'NONE', 'NONE',  #17 ) ;
#4381=EDGE_CURVE ( 'NONE', #10063, #17033, #16761, .T. ) ;
#4382=FACE_OUTER_BOUND ( 'NONE', #11513, .T. ) ;
#4397=CARTESIAN_POINT ( 'NONE',  ( -7.999999999629061165, -18.86445920977251234, -40.99220581062246538 ) ) ;
#4401=B_SPLINE_CURVE_WITH_KNOTS ( 'NONE', 3,
 ( #17712, #15214, #912, #27331, #5769, #757 ),
 .UNSPECIFIED., .F., .F.,
 ( 4, 2, 4 ),
 ( 0.000000000000000000, 0.5000000000000000000, 1.000000000000000000 ),
 .UNSPECIFIED. ) ;
#4405=EDGE_CURVE ( 'NONE', #6605, #27863, #11543, .T. ) ;
#4410=CARTESIAN_POINT ( 'NONE',  ( 8.700000000252410715, -24.26136093482726608, -29.62468611105379779 ) ) ;
#4416=ORIENTED_EDGE ( 'NONE', *, *, #14650, .T. ) ;
#4423=EDGE_CURVE ( 'NONE', #1748, #23469, #28453, .T. ) ;
#4442=ADVANCED_FACE ( 'NONE', ( #28884 ), #24316, .T. ) ;
#4452=CARTESIAN_POINT ( 'NONE',  ( 8.700000000241654874, -24.19757157926353486, -27.32949869323976699 ) ) ;
#4454=ORIENTED_EDGE ( 'NONE', *, *, #13252, .F. ) ;
#4458=VERTEX_POINT ( 'NONE', #2914 ) ;
#4460=SURFACE_SIDE_STYLE ('',( #11386 ) ) ;
#4462=EDGE_LOOP ( 'NONE', ( #27785, #11812, #28209, #9013 ) ) ;
#4472=EDGE_CURVE ( 'NONE', #5752, #7991, #21293, .T. ) ;
#4509=DIRECTION ( 'NONE',  ( 2.764802276011834743E-12, 0.9128796883888953273, -0.4082287037029531662 ) ) ;
#4513=CARTESIAN_POINT ( 'NONE',  ( 6.999999999945624829, -115.1185614904238577, 21.95989595801592031 ) ) ;
#4514=ORIENTED_EDGE ( 'NONE', *, *, #10467, .T. ) ;
#4516=CARTESIAN_POINT ( 'NONE',  ( -8.699999999650268379, -15.05691612485074948, -37.86814428179198444 ) ) ;
#4525=CARTESIAN_POINT ( 'NONE',  ( -7.999999999726708388, -29.41772009837547586, -26.57524823659570146 ) ) ;
#4543=CARTESIAN_POINT ( 'NONE',  ( 8.700000000252410715, -24.26136093482726608, -29.62468611105379779 ) ) ;
#4557=CARTESIAN_POINT ( 'NONE',  ( 8.700000000289984214, -14.75121143964889292, -37.75136796596272148 ) ) ;
#4567=ORIENTED_EDGE ( 'NONE', *, *, #3884, .T. ) ;
#4595=LINE ( 'NONE', #23344, #17284 ) ;
#4598=FACE_OUTER_BOUND ( 'NONE', #13478, .T. ) ;
#4601=EDGE_LOOP ( 'NONE', ( #17333, #23624, #15907, #25632, #10441, #8662, #12181, #21943 ) ) ;
#4616=ORIENTED_EDGE ( 'NONE', *, *, #17169, .F. ) ;
#4624=CARTESIAN_POINT ( 'NONE',  ( 8.000000000245886866, -28.22468611110216230, -31.13863906511491209 ) ) ;
#4636=CARTESIAN_POINT ( 'NONE',  ( -7.999999999661569383, -18.38684431933573649, -36.12071760317176228 ) ) ;
#4645=ORIENTED_EDGE ( 'NONE', *, *, #2333, .T. ) ;
#4658=LINE ( 'NONE', #16613, #16028 ) ;
#4667=CARTESIAN_POINT ( 'NONE',  ( 4.276011752548591005, -110.9401521129877892, -1.050525799503824409 ) ) ;
#4668=ADVANCED_FACE ( 'NONE', ( #20685 ), #4320, .T. ) ;
#4669=CARTESIAN_POINT ( 'NONE',  ( 8.700000000277906764, -15.94902145836247342, -35.53273252485295330 ) ) ;
#4677=ORIENTED_EDGE ( 'NONE', *, *, #28548, .F. ) ;
#4679=LINE ( 'NONE', #12376, #28318 ) ;
#4695=CARTESIAN_POINT ( 'NONE',  ( 8.700000000276881806, -18.45710910160467932, -35.79080037231529587 ) ) ;
#4703=CARTESIAN_POINT ( 'NONE',  ( -8.699999999697419995, -28.90937277432163199, -30.74718652567387522 ) ) ;
#4726=ORIENTED_EDGE ( 'NONE', *, *, #25225, .T. ) ;
#4731=DIRECTION ( 'NONE',  ( 1.000000000000000000, -1.843431230208684678E-12, 2.650498504958264790E-12 ) ) ;
#4749=FACE_OUTER_BOUND ( 'NONE', #26017, .T. ) ;
#4754=CARTESIAN_POINT ( 'NONE',  ( -8.000000000005952572, -116.8591659214701792, 11.34031266722930908 ) ) ;
#4757=APPLICATION_CONTEXT ( 'automotive_design' ) ;
#4795=VECTOR ( 'NONE', #4138, 999.9999999999998863 ) ;
#4797=LINE ( 'NONE', #6618, #1925 ) ;
#4837=CARTESIAN_POINT ( 'NONE',  ( -7.999999999729645594, -28.43173360601001320, -25.75874043427127091 ) ) ;
#4842=EDGE_CURVE ( 'NONE', #16921, #23754, #2879, .T. ) ;
#4852=ORIENTED_EDGE ( 'NONE', *, *, #27429, .F. ) ;
#4871=CARTESIAN_POINT ( 'NONE',  ( 8.699999999974050269, -116.8589940799748632, 11.34037320843244956 ) ) ;
#4891=EDGE_CURVE ( 'NONE', #23146, #2707, #14136, .T. ) ;
#4894=EDGE_CURVE ( 'NONE', #28185, #16, #383, .T. ) ;
#4903=DIRECTION ( 'NONE',  ( -1.000000000000000000, 5.687697999151106851E-16, -6.771501495036750356E-12 ) ) ;
#4910=DIRECTION ( 'NONE',  ( 1.000000000000000000, -1.843431230200084908E-12, 2.650498504963248473E-12 ) ) ;
#4943=CARTESIAN_POINT ( 'NONE',  ( 8.700000000279958456, -18.28438020625039329, -36.42481760783426381 ) ) ;
#4961=CARTESIAN_POINT ( 'NONE',  ( 8.000000000241653808, -24.19750966826863348, -27.32947504231146851 ) ) ;
#4964=CARTESIAN_POINT ( 'NONE',  ( -7.999999999639610948, -13.66761481655621147, -39.85825877797649497 ) ) ;
#4966=CARTESIAN_POINT ( 'NONE',  ( 8.700000000296645553, -12.00150950392997018, -38.75816838998848368 ) ) ;
#4971=PLANE ( 'NONE',  #450 ) ;
#5035=CYLINDRICAL_SURFACE ( 'NONE', #9454, 2.500000000000002220 ) ;
#5059=ORIENTED_EDGE ( 'NONE', *, *, #421, .T. ) ;
#5061=CARTESIAN_POINT ( 'NONE',  ( 8.000000000735305150, -25.09035620894639962, -26.05319937780492623 ) ) ;
#5065=PLANE ( 'NONE',  #19363 ) ;
#5066=FACE_OUTER_BOUND ( 'NONE', #13070, .T. ) ;
#5074=CARTESIAN_POINT ( 'NONE',  ( -8.699999999649984161, -14.75061022399014909, -37.75108774327986083 ) ) ;
#5075=CARTESIAN_POINT ( 'NONE',  ( -7.999999999682583685, -17.59928882257115390, -33.62871304529124927 ) ) ;
#5109=DIRECTION ( 'NONE',  ( -3.924189347185962345E-12, 0.4082287037029530552, 0.9128796883888953273 ) ) ;
#5113=CARTESIAN_POINT ( 'NONE',  ( -7.999999999648228055, -10.57732533965963384, -37.42446625050693854 ) ) ;
#5132=ORIENTED_EDGE ( 'NONE', *, *, #30437, .F. ) ;
#5180=CARTESIAN_POINT ( 'NONE',  ( -8.000000000477658801, -25.77531388886969310, -25.66136093485691916 ) ) ;
#5190=DIRECTION ( 'NONE',  ( -1.000000000000000000, 5.687697999151106851E-16, -6.771501495036750356E-12 ) ) ;
#5214=CARTESIAN_POINT ( 'NONE',  ( -7.999999999652283478, -16.96959321758620476, -37.81493174591201978 ) ) ;
#5217=PLANE ( 'NONE',  #7957 ) ;
#5225=CARTESIAN_POINT ( 'NONE',  ( -7.999999999719186405, -5.927479909175757733, -27.82023779336357094 ) ) ;
#5230=VECTOR ( 'NONE', #11561, 1000.000000000000000 ) ;
#5252=VERTEX_POINT ( 'NONE', #19376 ) ;
#5254=DIRECTION ( 'NONE',  ( 2.416122857340496113E-12, -0.9341647027306024809, -0.3568421334038978099 ) ) ;
#5266=ORIENTED_EDGE ( 'NONE', *, *, #12718, .T. ) ;
#5271=AXIS2_PLACEMENT_3D ( 'NONE', #9862, #19462, #29053 ) ;
#5280=CARTESIAN_POINT ( 'NONE',  ( -7.999999999681902452, -14.92844969907143771, -33.25053330396754347 ) ) ;
#5326=CARTESIAN_POINT ( 'NONE',  ( -7.999999999957778662, -114.8354788345922941, 7.878836663909118521 ) ) ;
#5343=CARTESIAN_POINT ( 'NONE',  ( -7.999999999727681832, -25.78362547594782583, -25.65764409411462310 ) ) ;
#5344=ORIENTED_EDGE ( 'NONE', *, *, #4249, .T. ) ;
#5357=ADVANCED_FACE ( 'NONE', ( #4749 ), #14354, .F. ) ;
#5362=CARTESIAN_POINT ( 'NONE',  ( -8.699999999728817102, -29.34680062185485738, -26.49035620860901474 ) ) ;
#5386=DIRECTION ( 'NONE',  ( -1.000000000000000000, 5.687697993419811493E-16, -6.771501495049272772E-12 ) ) ;
#5407=ORIENTED_EDGE ( 'NONE', *, *, #20120, .T. ) ;
#5418=ADVANCED_FACE ( 'NONE', ( #8594 ), #22936, .T. ) ;
#5444=ADVANCED_FACE ( 'NONE', ( #22196 ), #8758, .F. ) ;
#5472=CARTESIAN_POINT ( 'NONE',  ( 8.700000000276082446, -16.84110654130126150, -33.19737377701691372 ) ) ;
#5477=AXIS2_PLACEMENT_3D ( 'NONE', #17844, #25425, #15186 ) ;
#5482=ORIENTED_EDGE ( 'NONE', *, *, #6809, .F. ) ;
#5496=DIRECTION ( 'NONE',  ( 1.000000000000000000, -9.219999999999999084E-13, 4.710999999999999616E-12 ) ) ;
#5537=DIRECTION ( 'NONE',  ( -1.000000000000000000, -1.601966730286662369E-12, -3.582312748438143944E-12 ) ) ;
#5549=DIRECTION ( 'NONE',  ( 1.000000000000000000, -1.843431230200084908E-12, 2.650498504963248473E-12 ) ) ;
#5560=ORIENTED_EDGE ( 'NONE', *, *, #28306, .F. ) ;
#5583=DIRECTION ( 'NONE',  ( 1.000000000000000000, -1.843431230198065828E-12, 2.650498504953516580E-12 ) ) ;
#5591=CARTESIAN_POINT ( 'NONE',  ( -7.999999999674140660, -13.61361098168129224, -34.64062768038885309 ) ) ;
#5593=VECTOR ( 'NONE', #16392, 1000.000000000000000 ) ;
#5620=CARTESIAN_POINT ( 'NONE',  ( 8.000000000286558333, -7.565603753400573339, -31.48340496130054689 ) ) ;
#5628=EDGE_CURVE ( 'NONE', #23079, #21601, #22435, .T. ) ;
#5632=( GEOMETRIC_REPRESENTATION_CONTEXT ( 3 ) GLOBAL_UNCERTAINTY_ASSIGNED_CONTEXT ( ( #30485 ) ) GLOBAL_UNIT_ASSIGNED_CONTEXT ( ( #24196, #29213, #2638 ) ) REPRESENTATION_CONTEXT ( 'NONE', 'WORKASPACE' ) );
#5640=CARTESIAN_POINT ( 'NONE',  ( -8.699999999679551621, -14.62812833074668184, -33.38483337050165289 ) ) ;
#5666=CARTESIAN_POINT ( 'NONE',  ( -7.707106781243226123, -115.2381289094444128, 21.69251968763726879 ) ) ;
#5675=CARTESIAN_POINT ( 'NONE',  ( 8.700000000133357503, -67.40749995146175877, -17.04319545392437263 ) ) ;
#5680=ORIENTED_EDGE ( 'NONE', *, *, #27186, .T. ) ;
#5691=CARTESIAN_POINT ( 'NONE',  ( -7.707106507371444870, -5.692566414263196428, -27.29492500646317765 ) ) ;
#5698=CARTESIAN_POINT ( 'NONE',  ( -8.000000000444114079, -28.22468611108740788, -31.13863906519029001 ) ) ;
#5708=B_SPLINE_CURVE_WITH_KNOTS ( 'NONE', 3,
 ( #19725, #22087, #545, #28696, #10125, #21466 ),
 .UNSPECIFIED., .F., .F.,
 ( 4, 2, 4 ),
 ( 0.000000000000000000, 0.5000000000000000000, 1.000000000000000000 ),
 .UNSPECIFIED. ) ;
#5720=COLOUR_RGB ( '', 0.31764706, 0.68627451, 0.89019608) ;
#5732=ORIENTED_EDGE ( 'NONE', *, *, #4891, .T. ) ;
#5746=FACE_OUTER_BOUND ( 'NONE', #28008, .T. ) ;
#5752=VERTEX_POINT ( 'NONE', #8876 ) ;
#5757=VECTOR ( 'NONE', #21437, 1000.000000000000000 ) ;
#5769=CARTESIAN_POINT ( 'NONE',  ( 8.700000000279912271, -18.16707915929421446, -36.73187106089413589 ) ) ;
#5770=DIRECTION ( 'NONE',  ( -1.000000000000000000, 5.687698019339887572E-16, -6.771501495046482653E-12 ) ) ;
#5771=VECTOR ( 'NONE', #15372, 1000.000000000000000 ) ;
#5775=EDGE_CURVE ( 'NONE', #22456, #368, #25732, .T. ) ;
#5814=B_SPLINE_CURVE_WITH_KNOTS ( 'NONE', 5,
 ( #17636, #27248, #3021, #12613, #8188, #22225, #3323, #12928, #7885, #983, #10573, #25045 ),
 .UNSPECIFIED., .F., .F.,
 ( 6, 3, 3, 6 ),
 ( 2.782752057450000205, 3.293393370880000059, 4.940089941930000172, 5.565010780509999755 ),
 .UNSPECIFIED. ) ;
#5829=CARTESIAN_POINT ( 'NONE',  ( -7.999999999655180716, -13.66682223735657864, -36.55330428419717492 ) ) ;
#5830=CARTESIAN_POINT ( 'NONE',  ( 7.999488503669390127, -115.5102744061023543, 21.08394882064870401 ) ) ;
#5865=ORIENTED_EDGE ( 'NONE', *, *, #713, .F. ) ;
#5866=ORIENTED_EDGE ( 'NONE', *, *, #8704, .T. ) ;
#5894=DIRECTION ( 'NONE',  ( 1.000000000000000000, -1.843431230198065828E-12, 2.650498504953516580E-12 ) ) ;
#5906=CYLINDRICAL_SURFACE ( 'NONE', #31053, 1.000000000000000888 ) ;
#5927=EDGE_CURVE ( 'NONE', #1828, #4237, #14232, .T. ) ;
#5937=DIRECTION ( 'NONE',  ( 1.000000000000000000, -1.843431230208684678E-12, 2.650498504958264790E-12 ) ) ;
#5987=B_SPLINE_CURVE_WITH_KNOTS ( 'NONE', 5,
 ( #16472, #26086, #4525, #14123, #23731, #4837, #16779, #24492, #12214 ),
 .UNSPECIFIED., .F., .F.,
 ( 6, 3, 6 ),
 ( 0.000000000000000000, 2.405120303529999948, 3.339306057039999498 ),
 .UNSPECIFIED. ) ;
#6002=B_SPLINE_CURVE_WITH_KNOTS ( 'NONE', 5,
 ( #17944, #30080, #12933, #27707, #10577, #12782, #17641, #27254, #5691 ),
 .UNSPECIFIED., .F., .F.,
 ( 6, 3, 6 ),
 ( 0.000000000000000000, 0.6973066785939999734, 1.117931991880000142 ),
 .UNSPECIFIED. ) ;
#6025=ORIENTED_EDGE ( 'NONE', *, *, #4423, .T. ) ;
#6044=FACE_OUTER_BOUND ( 'NONE', #18135, .T. ) ;
#6051=CARTESIAN_POINT ( 'NONE',  ( 8.000000000270995670, -18.23122067931581114, -34.51216076560703527 ) ) ;
#6074=EDGE_CURVE ( 'NONE', #1905, #17033, #8360, .T. ) ;
#6080=VERTEX_POINT ( 'NONE', #17955 ) ;
#6085=CARTESIAN_POINT ( 'NONE',  ( -8.699999999660043670, -18.28443321518998133, -36.42483785847389299 ) ) ;
#6091=DIRECTION ( 'NONE',  ( 1.000000000000000000, -9.219545062029677348E-13, 4.710284450064082408E-12 ) ) ;
#6097=VERTEX_POINT ( 'NONE', #17805 ) ;
#6111=CARTESIAN_POINT ( 'NONE',  ( -8.699999999691694796, -25.92947359974585098, -31.20249410827203107 ) ) ;
#6125=DIRECTION ( 'NONE',  ( 1.000000000000000000, -1.843431230198065424E-12, 2.650498504953516580E-12 ) ) ;
#6143=ORIENTED_EDGE ( 'NONE', *, *, #29397, .F. ) ;
#6147=ORIENTED_EDGE ( 'NONE', *, *, #6885, .T. ) ;
#6157=ORIENTED_EDGE ( 'NONE', *, *, #10467, .F. ) ;
#6217=VECTOR ( 'NONE', #2, 1000.000000000000227 ) ;
#6232=EDGE_CURVE ( 'NONE', #19159, #2499, #31018, .T. ) ;
#6265=ORIENTED_EDGE ( 'NONE', *, *, #2619, .F. ) ;
#6271=EDGE_LOOP ( 'NONE', ( #9137, #25470, #19827, #22708 ) ) ;
#6276=SURFACE_SIDE_STYLE ('',( #13508 ) ) ;
#6279=CARTESIAN_POINT ( 'NONE',  ( 8.000000000839076364, -16.52148444845764885, -38.01532054216111334 ) ) ;
#6296=CARTESIAN_POINT ( 'NONE',  ( -8.699999999662320960, -13.45909514929641304, -35.92961830801370127 ) ) ;
#6329=CARTESIAN_POINT ( 'NONE',  ( -7.260640027187754697, -115.1289678868684803, 21.93662520831884066 ) ) ;
#6330=FACE_OUTER_BOUND ( 'NONE', #1432, .T. ) ;
#6348=FILL_AREA_STYLE_COLOUR ( '', #6768 ) ;
#6351=CARTESIAN_POINT ( 'NONE',  ( -8.699999999628824199, -19.62590121859827619, -40.87657246514151410 ) ) ;
#6359=CARTESIAN_POINT ( 'NONE',  ( 8.699999999974050269, -116.8589940799748632, 11.34037320843244956 ) ) ;
#6404=CARTESIAN_POINT ( 'NONE',  ( 2.746585479520242742E-10, -5.287238790993575854, -26.38853270457268607 ) ) ;
#6432=CARTESIAN_POINT ( 'NONE',  ( 8.000000000660609345, -13.38331437764704113, -35.60411298974170080 ) ) ;
#6437=AXIS2_PLACEMENT_3D ( 'NONE', #30816, #27984, #25794 ) ;
#6441=CARTESIAN_POINT ( 'NONE',  ( -8.000000000196104466, -28.90964379102386062, -30.74680062216425469 ) ) ;
#6442=DIRECTION ( 'NONE',  ( -2.764840495839172514E-12, -0.9128796883888952163, 0.4082287037029530552 ) ) ;
#6445=EDGE_CURVE ( 'NONE', #21330, #3666, #2432, .T. ) ;
#6446=CARTESIAN_POINT ( 'NONE',  ( 7.260640027522912376, -5.583405280045696806, -27.05081923603077243 ) ) ;
#6457=CARTESIAN_POINT ( 'NONE',  ( 8.700000000285857737, -13.61366271048277277, -34.64064744186795508 ) ) ;
#6463=VERTEX_POINT ( 'NONE', #26947 ) ;
#6468=CARTESIAN_POINT ( 'NONE',  ( 8.700000000278096834, -14.92844969908683517, -33.25053330388887218 ) ) ;
#6474=ADVANCED_FACE ( 'NONE', ( #26330, #9640, #14378 ), #24125, .F. ) ;
#6479=CARTESIAN_POINT ( 'NONE',  ( -7.707106781243226123, -115.2381289094444128, 21.69251968763726879 ) ) ;
#6480=LINE ( 'NONE', #26153, #5593 ) ;
#6504=CARTESIAN_POINT ( 'NONE',  ( -8.699999999650465554, -17.26991458595691142, -37.68063167936340108 ) ) ;
#6507=ADVANCED_FACE ( 'NONE', ( #26635 ), #7736, .F. ) ;
#6512=ORIENTED_EDGE ( 'NONE', *, *, #6232, .T. ) ;
#6531=EDGE_CURVE ( 'NONE', #22923, #6605, #12559, .T. ) ;
#6532=DIRECTION ( 'NONE',  ( 1.000000000000000000, -9.219999999999999084E-13, 4.710999999999999616E-12 ) ) ;
#6533=CARTESIAN_POINT ( 'NONE',  ( -8.699999999997119815, -117.4706889483893377, 13.80759369055796526 ) ) ;
#6552=CARTESIAN_POINT ( 'NONE',  ( 8.700000000236576270, -29.80249410823907752, -29.47052640017699687 ) ) ;
#6558=LINE ( 'NONE', #18368, #605 ) ;
#6568=DIRECTION ( 'NONE',  ( 2.415891560877031462E-12, -0.9341647027306021478, -0.3568421334038983650 ) ) ;
#6574=EDGE_LOOP ( 'NONE', ( #6808, #13904, #23389, #20459 ) ) ;
#6575=SHAPE_DEFINITION_REPRESENTATION ( #4378, #24039 ) ;
#6605=VERTEX_POINT ( 'NONE', #20012 ) ;
#6617=CARTESIAN_POINT ( 'NONE',  ( -4.276011752264103016, -42.94729992905724458, -9.547410993472157159 ) ) ;
#6618=CARTESIAN_POINT ( 'NONE',  ( -8.699999998940043611, -18.28443321518998133, -36.42483785847389299 ) ) ;
#6621=EDGE_CURVE ( 'NONE', #28198, #23146, #5814, .T. ) ;
#6639=CARTESIAN_POINT ( 'NONE',  ( 8.699999999499924641, -28.07052640022601864, -25.59750589169981438 ) ) ;
#6653=ORIENTED_EDGE ( 'NONE', *, *, #1113, .T. ) ;
#6661=CARTESIAN_POINT ( 'NONE',  ( -8.000000000444114079, -28.22468611108740788, -31.13863906519029001 ) ) ;
#6683=B_SPLINE_CURVE_WITH_KNOTS ( 'NONE', 3,
 ( #20839, #25722, #13750, #9024, #18622, #25879 ),
 .UNSPECIFIED., .F., .F.,
 ( 4, 2, 4 ),
 ( 0.000000000000000000, 0.5000000000000000000, 1.000000000000000000 ),
 .UNSPECIFIED. ) ;
#6721=EDGE_CURVE ( 'NONE', #28711, #25555, #15591, .T. ) ;
#6731=AXIS2_PLACEMENT_3D ( 'NONE', #13960, #19761, #22120 ) ;
#6739=EDGE_CURVE ( 'NONE', #13665, #24204, #18423, .T. ) ;
#6752=CARTESIAN_POINT ( 'NONE',  ( 8.000000000354901886, -27.70368077928761252, -25.45737431365605019 ) ) ;
#6755=CARTESIAN_POINT ( 'NONE',  ( -7.999999999628144565, -17.92644052945513522, -41.00309170034211093 ) ) ;
#6768=COLOUR_RGB ( '', 0.31764706, 0.68627451, 0.89019608) ;
#6769=ORIENTED_EDGE ( 'NONE', *, *, #13506, .T. ) ;
#6775=VERTEX_POINT ( 'NONE', #6617 ) ;
#6788=ORIENTED_EDGE ( 'NONE', *, *, #19672, .F. ) ;
#6799=CARTESIAN_POINT ( 'NONE',  ( -7.999999999884559898, -60.75400889059668685, -3.446705952702470377 ) ) ;
#6805=EDGE_CURVE ( 'NONE', #15932, #15963, #20946, .T. ) ;
#6808=ORIENTED_EDGE ( 'NONE', *, *, #20808, .T. ) ;
#6809=EDGE_CURVE ( 'NONE', #10105, #2499, #30550, .T. ) ;
#6816=DIRECTION ( 'NONE',  ( 1.000000000000000000, -1.843431230200084908E-12, 2.650498504963248473E-12 ) ) ;
#6836=DIRECTION ( 'NONE',  ( -3.924189347185962345E-12, 0.4082287037029530552, 0.9128796883888953273 ) ) ;
#6864=LINE ( 'NONE', #28890, #3714 ) ;
#6877=ORIENTED_EDGE ( 'NONE', *, *, #20808, .F. ) ;
#6879=EDGE_LOOP ( 'NONE', ( #6147, #20671, #13740, #28139 ) ) ;
#6882=CARTESIAN_POINT ( 'NONE',  ( -8.699999999977865883, -116.4387282385435185, 10.14683980286297604 ) ) ;
#6885=EDGE_CURVE ( 'NONE', #19970, #16882, #16993, .T. ) ;
#6920=ORIENTED_EDGE ( 'NONE', *, *, #13369, .F. ) ;
#6928=ORIENTED_EDGE ( 'NONE', *, *, #29196, .T. ) ;
#6936=DIRECTION ( 'NONE',  ( 6.326189572192215265E-12, 0.3568421334038983650, -0.9341647027306021478 ) ) ;
#6989=CARTESIAN_POINT ( 'NONE',  ( 8.699999999528305494, -25.92947359976189503, -31.20249410819006286 ) ) ;
#6995=EDGE_CURVE ( 'NONE', #30810, #17596, #10539, .T. ) ;
#7030=CARTESIAN_POINT ( 'NONE',  ( 8.700000000232158470, -29.34712076613124410, -26.49064271397861603 ) ) ;
#7051=CARTESIAN_POINT ( 'NONE',  ( -8.699999999628362346, -14.95623164695839513, -40.37561726986208299 ) ) ;
#7052=CARTESIAN_POINT ( 'NONE',  ( -8.699999999662093586, -15.94902145834643115, -35.53273252493492862 ) ) ;
#7055=CARTESIAN_POINT ( 'NONE',  ( -6.999999999888483870, -60.34578018689466461, -2.533826264308865817 ) ) ;
#7069=CYLINDRICAL_SURFACE ( 'NONE', #28788, 2.500000000000002220 ) ;
#7070=DIRECTION ( 'NONE',  ( -6.325958275728752229E-12, -0.3568421334038983650, 0.9341647027306021478 ) ) ;
#7072=EDGE_CURVE ( 'NONE', #31008, #30761, #14558, .T. ) ;
#7077=CARTESIAN_POINT ( 'NONE',  ( 8.700000000244115128, -26.99999999999395328, -28.39999999994493862 ) ) ;
#7078=CARTESIAN_POINT ( 'NONE',  ( -7.999999999650399651, -14.92320859811129097, -37.81428931786641812 ) ) ;
#7084=ORIENTED_EDGE ( 'NONE', *, *, #15610, .F. ) ;
#7099=B_SPLINE_CURVE_WITH_KNOTS ( 'NONE', 3,
 ( #6661, #8703, #20517, #18310, #11083, #18145 ),
 .UNSPECIFIED., .F., .F.,
 ( 4, 2, 4 ),
 ( 0.000000000000000000, 0.5000000000000000000, 1.000000000000000000 ),
 .UNSPECIFIED. ) ;
#7113=EDGE_LOOP ( 'NONE', ( #27133, #2821, #5732, #20429 ) ) ;
#7114=CARTESIAN_POINT ( 'NONE',  ( 8.700000000276082446, -16.84110654130126150, -33.19737377701691372 ) ) ;
#7119=ORIENTED_EDGE ( 'NONE', *, *, #19079, .T. ) ;
#7127=CARTESIAN_POINT ( 'NONE',  ( -7.999999999718669486, -5.981227587262960554, -27.94042817487965991 ) ) ;
#7128=ORIENTED_EDGE ( 'NONE', *, *, #14968, .F. ) ;
#7147=DIRECTION ( 'NONE',  ( 2.415891560877031462E-12, -0.9341647027306021478, -0.3568421334038983650 ) ) ;
#7150=DIRECTION ( 'NONE',  ( 7.764622278472185525E-13, 0.9341647027306024809, 0.3568421334038978099 ) ) ;
#7154=CARTESIAN_POINT ( 'NONE',  ( -7.999999999660042604, -18.28443193496838504, -36.42483736938474692 ) ) ;
#7192=ORIENTED_EDGE ( 'NONE', *, *, #20888, .F. ) ;
#7239=ORIENTED_EDGE ( 'NONE', *, *, #402, .F. ) ;
#7258=AXIS2_PLACEMENT_3D ( 'NONE', #23955, #11975, #34 ) ;
#7261=AXIS2_PLACEMENT_3D ( 'NONE', #10354, #3259, #27181 ) ;
#7275=CARTESIAN_POINT ( 'NONE',  ( 7.000000000115440102, -60.75400889061052112, -3.446705952631804681 ) ) ;
#7276=CARTESIAN_POINT ( 'NONE',  ( 8.000000000284819279, -13.66682223737133128, -36.55330428412179344 ) ) ;
#7288=DIRECTION ( 'NONE',  ( -2.764840495839172918E-12, -0.9128796883888953273, 0.4082287037029531107 ) ) ;
#7298=CARTESIAN_POINT ( 'NONE',  ( -7.999999999650683868, -16.30392683535412957, -38.02387007715461920 ) ) ;
#7317=EDGE_CURVE ( 'NONE', #16606, #6097, #2178, .T. ) ;
#7333=CARTESIAN_POINT ( 'NONE',  ( -8.000000000002907896, -107.4273096626132116, 14.66297538107212262 ) ) ;
#7343=DIRECTION ( 'NONE',  ( -3.924189347185961537E-12, 0.4082287037029530552, 0.9128796883888952163 ) ) ;
#7347=EDGE_CURVE ( 'NONE', #18002, #30101, #26200, .T. ) ;
#7366=DIRECTION ( 'NONE',  ( 1.000000000000000000, -1.843431230208684274E-12, 2.650498504958264790E-12 ) ) ;
#7378=CARTESIAN_POINT ( 'NONE',  ( -7.999999999985950794, -116.8591659214701792, 11.34031266722930908 ) ) ;
#7393=CARTESIAN_POINT ( 'NONE',  ( -7.999999999730326827, -27.67628966639927057, -25.46613455157947570 ) ) ;
#7435=CARTESIAN_POINT ( 'NONE',  ( -7.999999999683784502, -16.99089124002251694, -33.25453181222756882 ) ) ;
#7436=EDGE_CURVE ( 'NONE', #3834, #30810, #30630, .T. ) ;
#7481=CARTESIAN_POINT ( 'NONE',  ( -8.350000000008115819, -22.83323352208430634, -39.84673050100227698 ) ) ;
#7486=CARTESIAN_POINT ( 'NONE',  ( 8.700000000289733748, -15.05693637256081097, -37.86809127166881694 ) ) ;
#7491=LINE ( 'NONE', #4667, #2651 ) ;
#7510=DIRECTION ( 'NONE',  ( 1.000000000000000000, -9.224647189900196894E-13, 4.710284450064082408E-12 ) ) ;
#7515=DIRECTION ( 'NONE',  ( -2.416122857340496113E-12, 0.9341647027306024809, 0.3568421334038978099 ) ) ;
#7525=VECTOR ( 'NONE', #25518, 1000.000000000000000 ) ;
#7545=ORIENTED_EDGE ( 'NONE', *, *, #4842, .T. ) ;
#7589=CARTESIAN_POINT ( 'NONE',  ( -7.999999999683340413, -17.27538706577754724, -33.40447746430434961 ) ) ;
#7593=CARTESIAN_POINT ( 'NONE',  ( 8.000000000276081380, -16.84112630282697154, -33.19732204816383359 ) ) ;
#7604=CARTESIAN_POINT ( 'NONE',  ( 8.000000000651317222, -14.08431897228786411, -33.76897726028251157 ) ) ;
#7608=ORIENTED_EDGE ( 'NONE', *, *, #14635, .F. ) ;
#7641=CARTESIAN_POINT ( 'NONE',  ( 2.774054804950544682E-10, -5.572998883585641217, -27.02754848644491403 ) ) ;
#7644=EDGE_CURVE ( 'NONE', #9163, #11537, #6683, .T. ) ;
#7664=EDGE_LOOP ( 'NONE', ( #26321, #30322, #26418, #23205 ) ) ;
#7670=VECTOR ( 'NONE', #5549, 1000.000000000000000 ) ;
#7677=CARTESIAN_POINT ( 'NONE',  ( 8.699999999966381736, -117.4706889487312083, 13.80759369670018444 ) ) ;
#7680=VERTEX_POINT ( 'NONE', #7593 ) ;
#7683=ADVANCED_FACE ( 'NONE', ( #2420 ), #10275, .T. ) ;
#7688=ORIENTED_EDGE ( 'NONE', *, *, #12089, .T. ) ;
#7693=CARTESIAN_POINT ( 'NONE',  ( -7.999999999727729794, -25.80029109889006023, -25.65030496461561071 ) ) ;
#7722=CARTESIAN_POINT ( 'NONE',  ( 8.000000000241653808, -24.19750966826863348, -27.32947504231146851 ) ) ;
#7726=CARTESIAN_POINT ( 'NONE',  ( -8.699999999693083907, -27.47644226430233871, -31.38783462183295114 ) ) ;
#7730=VERTEX_POINT ( 'NONE', #14847 ) ;
#7736=CYLINDRICAL_SURFACE ( 'NONE', #18325, 4.276011752367103291 ) ;
#7814=PLANE ( 'NONE',  #4003 ) ;
#7815=EDGE_CURVE ( 'NONE', #9796, #21330, #6002, .T. ) ;
#7819=FACE_OUTER_BOUND ( 'NONE', #14104, .T. ) ;
#7831=CARTESIAN_POINT ( 'NONE',  ( 7.000000000281329626, -5.981227587276792157, -27.94042817480899288 ) ) ;
#7859=B_SPLINE_CURVE_WITH_KNOTS ( 'NONE', 4,
 ( #17051, #26650, #7604, #24451, #28701 ),
 .UNSPECIFIED., .F., .F.,
 ( 5, 5 ),
 ( -0.9817477042469999748, 0.9817477042469999748 ),
 .UNSPECIFIED. ) ;
#7861=ADVANCED_FACE ( 'NONE', ( #29923 ), #3634, .F. ) ;
#7870=ORIENTED_EDGE ( 'NONE', *, *, #3586, .F. ) ;
#7885=CARTESIAN_POINT ( 'NONE',  ( -7.999999999653060634, -17.20645473190809227, -37.69618843468767722 ) ) ;
#7922=CARTESIAN_POINT ( 'NONE',  ( -7.999999999985950794, -116.8591659214701792, 11.34031266722930908 ) ) ;
#7944=AXIS2_PLACEMENT_3D ( 'NONE', #20207, #29958, #22890 ) ;
#7952=CARTESIAN_POINT ( 'NONE',  ( 8.700000000244115128, -26.99999999999395328, -28.39999999994493862 ) ) ;
#7955=CARTESIAN_POINT ( 'NONE',  ( -6.999999999884560786, -60.75400889059761766, -3.446705952697758590 ) ) ;
#7957=AXIS2_PLACEMENT_3D ( 'NONE', #15435, #29600, #18250 ) ;
#7991=VERTEX_POINT ( 'NONE', #30520 ) ;
#7999=ORIENTED_EDGE ( 'NONE', *, *, #29496, .T. ) ;
#8005=VECTOR ( 'NONE', #11432, 1000.000000000000000 ) ;
#8007=DIRECTION ( 'NONE',  ( -2.764840495839172918E-12, -0.9128796883888953273, 0.4082287037029530552 ) ) ;
#8024=CARTESIAN_POINT ( 'NONE',  ( 8.000000000229924524, -28.07052495763006661, -25.59750966822355522 ) ) ;
#8037=VERTEX_POINT ( 'NONE', #9099 ) ;
#8048=CARTESIAN_POINT ( 'NONE',  ( -7.999999999657077865, -13.50174601094418669, -36.11802512054224223 ) ) ;
#8083=ORIENTED_EDGE ( 'NONE', *, *, #4894, .T. ) ;
#8089=CARTESIAN_POINT ( 'NONE',  ( 8.699999999944495244, -116.0414483704658579, 19.89613934358818170 ) ) ;
#8144=ORIENTED_EDGE ( 'NONE', *, *, #9999, .F. ) ;
#8152=PLANE ( 'NONE',  #8407 ) ;
#8153=CARTESIAN_POINT ( 'NONE',  ( 8.000000000659929000, -16.02040192323402223, -38.09843960558792730 ) ) ;
#8164=CARTESIAN_POINT ( 'NONE',  ( -6.999999999891231006, -60.06002009430259392, -1.894810482436639409 ) ) ;
#8165=CARTESIAN_POINT ( 'NONE',  ( -7.800204957127538030, -115.2761342570987466, 21.60753225385484200 ) ) ;
#8172=ORIENTED_EDGE ( 'NONE', *, *, #25238, .T. ) ;
#8175=ORIENTED_EDGE ( 'NONE', *, *, #29212, .F. ) ;
#8178=CARTESIAN_POINT ( 'NONE',  ( -7.999999999694088260, -25.22378963202354996, -30.84934466693886534 ) ) ;
#8179=CARTESIAN_POINT ( 'NONE',  ( -8.699999999693680763, -27.86541989007905329, -31.29929855357051949 ) ) ;
#8184=VERTEX_POINT ( 'NONE', #4543 ) ;
#8188=CARTESIAN_POINT ( 'NONE',  ( -7.999999999657623206, -18.06128338792058230, -36.89507724070023897 ) ) ;
#8189=ORIENTED_EDGE ( 'NONE', *, *, #6739, .T. ) ;
#8216=EDGE_CURVE ( 'NONE', #11991, #9796, #21853, .T. ) ;
#8221=ORIENTED_EDGE ( 'NONE', *, *, #15029, .F. ) ;
#8255=ADVANCED_FACE ( 'NONE', ( #21538 ), #17111, .F. ) ;
#8261=CARTESIAN_POINT ( 'NONE',  ( -8.699999999715885224, -26.99999999997790923, -28.40000000002690683 ) ) ;
#8279=CARTESIAN_POINT ( 'NONE',  ( -8.699999999737658030, -25.77531388886905006, -25.66136093486021608 ) ) ;
#8289=EDGE_CURVE ( 'NONE', #24204, #25555, #19898, .T. ) ;
#8300=ORIENTED_EDGE ( 'NONE', *, *, #30470, .F. ) ;
#8318=CARTESIAN_POINT ( 'NONE',  ( -8.699999999638116321, -22.83323352287542463, -39.84673049988318638 ) ) ;
#8360=LINE ( 'NONE', #3036, #16792 ) ;
#8367=ORIENTED_EDGE ( 'NONE', *, *, #13800, .T. ) ;
#8374=ADVANCED_FACE ( 'NONE', ( #7819 ), #914, .F. ) ;
#8378=ORIENTED_EDGE ( 'NONE', *, *, #1443, .F. ) ;
#8386=CARTESIAN_POINT ( 'NONE',  ( 8.699999999991231192, -113.1082736041627896, 6.336644015525963347 ) ) ;
#8391=CARTESIAN_POINT ( 'NONE',  ( -8.699999998971694737, -25.92947359974585098, -31.20249410827203107 ) ) ;
#8405=LINE ( 'NONE', #30463, #10608 ) ;
#8407=AXIS2_PLACEMENT_3D ( 'NONE', #2989, #13187, #5496 ) ;
#8417=CARTESIAN_POINT ( 'NONE',  ( -8.699999999731330647, -26.52402217114853755, -25.41208138081151091 ) ) ;
#8419=CARTESIAN_POINT ( 'NONE',  ( 8.700000000294114244, -16.25281683561194868, -40.75997113242387826 ) ) ;
#8422=FACE_BOUND ( 'NONE', #4601, .T. ) ;
#8437=FACE_BOUND ( 'NONE', #12610, .T. ) ;
#8439=FACE_OUTER_BOUND ( 'NONE', #16245, .T. ) ;
#8441=CIRCLE ( 'NONE', #10982, 10.00000000000000178 ) ;
#8446=B_SPLINE_CURVE_WITH_KNOTS ( 'NONE', 3,
 ( #10104, #8179, #7726, #17332, #19862, #26938 ),
 .UNSPECIFIED., .F., .F.,
 ( 4, 2, 4 ),
 ( 0.000000000000000000, 0.5000000000000000000, 1.000000000000000000 ),
 .UNSPECIFIED. ) ;
#8478=FACE_OUTER_BOUND ( 'NONE', #12410, .T. ) ;
#8485=ORIENTED_EDGE ( 'NONE', *, *, #25123, .F. ) ;
#8506=CARTESIAN_POINT ( 'NONE',  ( -8.699999999650268379, -15.05691612485074948, -37.86814428179198444 ) ) ;
#8523=ORIENTED_EDGE ( 'NONE', *, *, #16365, .F. ) ;
#8549=CARTESIAN_POINT ( 'NONE',  ( 8.699999999987257482, -114.1237136972522990, 7.129097341238439967 ) ) ;
#8555=ORIENTED_EDGE ( 'NONE', *, *, #5775, .F. ) ;
#8565=ORIENTED_EDGE ( 'NONE', *, *, #1020, .F. ) ;
#8580=ORIENTED_EDGE ( 'NONE', *, *, #20258, .F. ) ;
#8594=FACE_OUTER_BOUND ( 'NONE', #30347, .T. ) ;
#8614=VECTOR ( 'NONE', #17721, 1000.000000000000000 ) ;
#8617=ORIENTED_EDGE ( 'NONE', *, *, #2913, .F. ) ;
#8662=ORIENTED_EDGE ( 'NONE', *, *, #18864, .F. ) ;
#8663=CARTESIAN_POINT ( 'NONE',  ( 7.999999999949441332, -116.5561065468434947, 18.74526241744673172 ) ) ;
#8673=LINE ( 'NONE', #3968, #24073 ) ;
#8679=CARTESIAN_POINT ( 'NONE',  ( 4.276011752472853367, -103.0613381315207988, 16.56805218640185018 ) ) ;
#8703=CARTESIAN_POINT ( 'NONE',  ( -7.999999999693026886, -27.86619909554637786, -31.29895010234936947 ) ) ;
#8704=EDGE_CURVE ( 'NONE', #2756, #15244, #13974, .T. ) ;
#8720=CARTESIAN_POINT ( 'NONE',  ( 8.700000000236576270, -29.80249410823907752, -29.47052640017699687 ) ) ;
#8742=ORIENTED_EDGE ( 'NONE', *, *, #16365, .T. ) ;
#8758=CYLINDRICAL_SURFACE ( 'NONE', #21839, 2.500000000000001776 ) ;
#8759=CYLINDRICAL_SURFACE ( 'NONE', #15261, 3.000000000000002220 ) ;
#8780=ORIENTED_EDGE ( 'NONE', *, *, #3399, .T. ) ;
#8783=PRESENTATION_STYLE_ASSIGNMENT (( #20748 ) ) ;
#8797=CARTESIAN_POINT ( 'NONE',  ( -4.276011752264103016, -102.7755780389424416, 17.20706796824344309 ) ) ;
#8802=CARTESIAN_POINT ( 'NONE',  ( 8.700000000232341435, -25.77531388888509056, -25.66136093477824431 ) ) ;
#8818=DIRECTION ( 'NONE',  ( -1.000000000000000000, 5.687697999151106851E-16, -6.771501495036750356E-12 ) ) ;
#8825=CARTESIAN_POINT ( 'NONE',  ( -8.699999999648019511, -15.69115814626919914, -38.04095234954149873 ) ) ;
#8836=DIRECTION ( 'NONE',  ( -3.924189347185962345E-12, 0.4082287037029531107, 0.9128796883888953273 ) ) ;
#8842=VERTEX_POINT ( 'NONE', #31117 ) ;
#8848=ADVANCED_FACE ( 'NONE', ( #26697 ), #14601, .F. ) ;
#8858=CARTESIAN_POINT ( 'NONE',  ( -8.699999999656894190, -18.16737667679718626, -36.73114375906605744 ) ) ;
#8865=DIRECTION ( 'NONE',  ( -8.077935669463159094E-28, -0.9128796883888953273, 0.4082287037029530552 ) ) ;
#8876=CARTESIAN_POINT ( 'NONE',  ( 8.700000000301640668, -14.95611408989196711, -40.37595097046296644 ) ) ;
#8905=CARTESIAN_POINT ( 'NONE',  ( 8.000000000264140709, -18.27877680372071723, -30.94409471150577318 ) ) ;
#8911=VERTEX_POINT ( 'NONE', #17701 ) ;
#8920=B_SPLINE_CURVE_WITH_KNOTS ( 'NONE', 3,
 ( #15896, #25499, #23144, #28472, #1891, #23294 ),
 .UNSPECIFIED., .F., .F.,
 ( 4, 2, 4 ),
 ( 0.000000000000000000, 0.5000000000000000000, 1.000000000000000000 ),
 .UNSPECIFIED. ) ;
#8922=CYLINDRICAL_SURFACE ( 'NONE', #26183, 10.00000000000000178 ) ;
#8930=ADVANCED_FACE ( 'NONE', ( #22450 ), #5906, .F. ) ;
#8957=CARTESIAN_POINT ( 'NONE',  ( 8.000000000856587690, -26.13380090421571111, -25.50104989771282149 ) ) ;
#9004=ORIENTED_EDGE ( 'NONE', *, *, #18821, .F. ) ;
#9005=CARTESIAN_POINT ( 'NONE',  ( 8.700000000278096834, -14.92844969908683517, -33.25053330388887218 ) ) ;
#9013=ORIENTED_EDGE ( 'NONE', *, *, #12551, .F. ) ;
#9023=CYLINDRICAL_SURFACE ( 'NONE', #29226, 3.000000000000002220 ) ;
#9024=CARTESIAN_POINT ( 'NONE',  ( 8.000000000735605354, -29.98791861930862268, -27.92402217156406152 ) ) ;
#9099=CARTESIAN_POINT ( 'NONE',  ( 8.700000000245887932, -28.22468611110281245, -31.13863906511161517 ) ) ;
#9113=CARTESIAN_POINT ( 'NONE',  ( 7.132997404352039439, -5.572998883428931904, -27.02754848604616456 ) ) ;
#9121=VERTEX_POINT ( 'NONE', #28866 ) ;
#9124=ORIENTED_EDGE ( 'NONE', *, *, #11822, .F. ) ;
#9126=ORIENTED_EDGE ( 'NONE', *, *, #6809, .T. ) ;
#9137=ORIENTED_EDGE ( 'NONE', *, *, #27518, .F. ) ;
#9138=AXIS2_PLACEMENT_3D ( 'NONE', #18197, #15683, #25294 ) ;
#9143=ADVANCED_FACE ( 'NONE', ( #21794 ), #23855, .T. ) ;
#9155=FACE_OUTER_BOUND ( 'NONE', #13715, .T. ) ;
#9163=VERTEX_POINT ( 'NONE', #19431 ) ;
#9166=CARTESIAN_POINT ( 'NONE',  ( -8.699999999660043670, -18.28443321518998133, -36.42483785847389299 ) ) ;
#9189=CARTESIAN_POINT ( 'NONE',  ( 1.030019577584204020E-10, -102.7755780389355778, 17.20706796825876239 ) ) ;
#9190=CARTESIAN_POINT ( 'NONE',  ( 8.000000000248304488, -25.92947504235655032, -31.20249033167290165 ) ) ;
#9207=ORIENTED_EDGE ( 'NONE', *, *, #6531, .F. ) ;
#9213=CARTESIAN_POINT ( 'NONE',  ( 8.700000000240452280, -29.66169484525095612, -29.83890322678064777 ) ) ;
#9258=CARTESIAN_POINT ( 'NONE',  ( -8.699999999694114194, -28.22468611108677194, -31.13863906519358693 ) ) ;
#9264=CARTESIAN_POINT ( 'NONE',  ( -7.999999999634344938, -21.57658477890130655, -40.40133997131670185 ) ) ;
#9278=( GEOMETRIC_REPRESENTATION_CONTEXT ( 3 ) GLOBAL_UNCERTAINTY_ASSIGNED_CONTEXT ( ( #2150 ) ) GLOBAL_UNIT_ASSIGNED_CONTEXT ( ( #3991, #18302, #23512 ) ) REPRESENTATION_CONTEXT ( 'NONE', 'WORKASPACE' ) );
#9287=VECTOR ( 'NONE', #4367, 999.9999999999998863 ) ;
#9289=AXIS2_PLACEMENT_3D ( 'NONE', #30540, #25348, #15579 ) ;
#9305=CARTESIAN_POINT ( 'NONE',  ( -7.132997404018626142, -115.1185614902475436, 21.95989595831449748 ) ) ;
#9306=DIRECTION ( 'NONE',  ( -2.764840495839172918E-12, -0.9128796883888953273, 0.4082287037029531107 ) ) ;
#9319=CARTESIAN_POINT ( 'NONE',  ( 8.699999999505822146, -29.73863906516063693, -27.17531388883607590 ) ) ;
#9324=ORIENTED_EDGE ( 'NONE', *, *, #28426, .F. ) ;
#9327=ADVANCED_FACE ( 'NONE', ( #20355 ), #29645, .T. ) ;
#9329=CARTESIAN_POINT ( 'NONE',  ( -8.699999999656061078, -13.80112230385522487, -36.85362565245412725 ) ) ;
#9348=ORIENTED_EDGE ( 'NONE', *, *, #9999, .T. ) ;
#9360=LINE ( 'NONE', #16602, #15425 ) ;
#9422=CARTESIAN_POINT ( 'NONE',  ( 7.505215711137140033, -5.625030866512529037, -27.14390223597047935 ) ) ;
#9426=ORIENTED_EDGE ( 'NONE', *, *, #2913, .T. ) ;
#9454=AXIS2_PLACEMENT_3D ( 'NONE', #14490, #4731, #16676 ) ;
#9470=ORIENTED_EDGE ( 'NONE', *, *, #19531, .T. ) ;
#9471=EDGE_CURVE ( 'NONE', #19001, #26338, #30705, .T. ) ;
#9500=EDGE_CURVE ( 'NONE', #30761, #23469, #23359, .T. ) ;
#9510=CIRCLE ( 'NONE', #5477, 4.276011752367109509 ) ;
#9553=CARTESIAN_POINT ( 'NONE',  ( 7.097978820185624649, -115.1185614902606744, 21.95989595838153718 ) ) ;
#9554=ORIENTED_EDGE ( 'NONE', *, *, #15634, .T. ) ;
#9557=ORIENTED_EDGE ( 'NONE', *, *, #4842, .F. ) ;
#9559=ADVANCED_FACE ( 'NONE', ( #23973 ), #21451, .T. ) ;
#9564=VECTOR ( 'NONE', #16030, 1000.000000000000114 ) ;
#9571=B_SPLINE_CURVE_WITH_KNOTS ( 'NONE', 3,
 ( #23240, #11120, #14107, #25448, #11587, #18357 ),
 .UNSPECIFIED., .F., .F.,
 ( 4, 2, 4 ),
 ( 0.000000000000000000, 0.5000000000000000000, 1.000000000000000000 ),
 .UNSPECIFIED. ) ;
#9574=DIRECTION ( 'NONE',  ( 3.134067079931429195E-12, 0.3568421334038983650, -0.9341647027306021478 ) ) ;
#9577=VERTEX_POINT ( 'NONE', #26631 ) ;
#9603=EDGE_LOOP ( 'NONE', ( #20311, #9124, #1361, #9716 ) ) ;
#9639=CARTESIAN_POINT ( 'NONE',  ( -8.699999999655181782, -13.66682223737418944, -36.55330428419230060 ) ) ;
#9640=FACE_BOUND ( 'NONE', #19323, .T. ) ;
#9641=ORIENTED_EDGE ( 'NONE', *, *, #9500, .T. ) ;
#9652=CARTESIAN_POINT ( 'NONE',  ( -7.999999999652283478, -16.96959321758620476, -37.81493174591201978 ) ) ;
#9658=FACE_OUTER_BOUND ( 'NONE', #7664, .T. ) ;
#9676=ORIENTED_EDGE ( 'NONE', *, *, #13956, .F. ) ;
#9687=DIRECTION ( 'NONE',  ( 2.249415931299125355E-12, -0.9431856258987900699, -0.3322662713817151059 ) ) ;
#9699=FACE_OUTER_BOUND ( 'NONE', #11530, .T. ) ;
#9709=CARTESIAN_POINT ( 'NONE',  ( 1.814857447021396585E-10, -110.9401521129946389, -1.050525799519145487 ) ) ;
#9714=CARTESIAN_POINT ( 'NONE',  ( 8.700000000234501485, -26.52350767672318810, -25.41191590392901034 ) ) ;
#9716=ORIENTED_EDGE ( 'NONE', *, *, #18462, .T. ) ;
#9735=CARTESIAN_POINT ( 'NONE',  ( 8.000000000829070146, -18.03083188300961481, -34.06405199645556792 ) ) ;
#9755=CARTESIAN_POINT ( 'NONE',  ( 8.699999999994835420, -111.9817663798902885, 5.760339591779549018 ) ) ;
#9761=B_SPLINE_CURVE_WITH_KNOTS ( 'NONE', 4,
 ( #17910, #15557, #25167, #11324, #18395 ),
 .UNSPECIFIED., .F., .F.,
 ( 5, 5 ),
 ( -0.9817477042469999748, 0.9817477042469999748 ),
 .UNSPECIFIED. ) ;
#9784=CARTESIAN_POINT ( 'NONE',  ( 8.000000000235820252, -29.73863906515999389, -27.17531388883937993 ) ) ;
#9796=VERTEX_POINT ( 'NONE', #1599 ) ;
#9799=DIRECTION ( 'NONE',  ( -8.579942312181285869E-13, -0.9431856258987900699, -0.3322662713817151059 ) ) ;
#9836=EDGE_CURVE ( 'NONE', #23146, #26338, #13705, .T. ) ;
#9843=CARTESIAN_POINT ( 'NONE',  ( -7.999999999664561656, -9.529422221863875109, -35.87488938007345496 ) ) ;
#9845=CARTESIAN_POINT ( 'NONE',  ( 8.700000000301640668, -14.95611408989196711, -40.37595097046296644 ) ) ;
#9862=CARTESIAN_POINT ( 'NONE',  ( 8.700000000244115128, -26.99999999999395328, -28.39999999994493862 ) ) ;
#9868=VERTEX_POINT ( 'NONE', #9755 ) ;
#9890=CARTESIAN_POINT ( 'NONE',  ( -8.699999999700381181, -24.65270539047089926, -30.30942439802224442 ) ) ;
#9891=ADVANCED_FACE ( 'NONE', ( #17139 ), #5035, .F. ) ;
#9898=CARTESIAN_POINT ( 'NONE',  ( 8.000000000456484628, -17.29968381802795463, -33.37248524067440769 ) ) ;
#9910=ORIENTED_EDGE ( 'NONE', *, *, #22783, .T. ) ;
#9920=CARTESIAN_POINT ( 'NONE',  ( 8.699999999531884853, -22.83323352251082738, -39.84673050073825351 ) ) ;
#9967=EDGE_CURVE ( 'NONE', #10105, #15932, #23185, .T. ) ;
#9974=AXIS2_PLACEMENT_3D ( 'NONE', #21342, #23711, #25915 ) ;
#9997=CARTESIAN_POINT ( 'NONE',  ( 8.700000000238844677, -25.09064271401819113, -26.05287923382458004 ) ) ;
#9999=EDGE_CURVE ( 'NONE', #2499, #15963, #12312, .T. ) ;
#10000=CARTESIAN_POINT ( 'NONE',  ( -7.999999999640660775, -13.05987697124905367, -39.51663027436784148 ) ) ;
#10003=AXIS2_PLACEMENT_3D ( 'NONE', #20731, #18036, #18369 ) ;
#10046=FACE_OUTER_BOUND ( 'NONE', #30019, .T. ) ;
#10056=CARTESIAN_POINT ( 'NONE',  ( -7.999999999949641172, -113.1810333093661995, 6.475256412746450252 ) ) ;
#10058=CARTESIAN_POINT ( 'NONE',  ( 8.699999999970108533, -117.2796036033498268, 12.53378553140980323 ) ) ;
#10063=VERTEX_POINT ( 'NONE', #21178 ) ;
#10079=EDGE_CURVE ( 'NONE', #3666, #4458, #9360, .T. ) ;
#10101=B_SPLINE_CURVE_WITH_KNOTS ( 'NONE', 3,
 ( #4624, #11865, #31064, #21625, #1968, #23991 ),
 .UNSPECIFIED., .F., .F.,
 ( 4, 2, 4 ),
 ( 0.000000000000000000, 0.5000000000000000000, 1.000000000000000000 ),
 .UNSPECIFIED. ) ;
#10104=CARTESIAN_POINT ( 'NONE',  ( -8.699999999694114194, -28.22468611108677194, -31.13863906519358693 ) ) ;
#10105=VERTEX_POINT ( 'NONE', #18651 ) ;
#10112=CARTESIAN_POINT ( 'NONE',  ( 8.700000000247854359, -24.42167197180108573, -29.98317312617670538 ) ) ;
#10125=CARTESIAN_POINT ( 'NONE',  ( -8.699999999708559528, -29.94314889530440738, -29.10209438447943953 ) ) ;
#10126=B_SPLINE_CURVE_WITH_KNOTS ( 'NONE', 3,
 ( #7114, #23656, #11682, #13733, #21282, #9005 ),
 .UNSPECIFIED., .F., .F.,
 ( 4, 2, 4 ),
 ( 0.000000000000000000, 0.4999999999999986677, 1.000000000000000000 ),
 .UNSPECIFIED. ) ;
#10156=CARTESIAN_POINT ( 'NONE',  ( -7.999999999683791607, -15.80258142959463363, -33.02070610725625954 ) ) ;
#10159=ORIENTED_EDGE ( 'NONE', *, *, #16817, .T. ) ;
#10161=CARTESIAN_POINT ( 'NONE',  ( 8.700000000288625301, -16.67085403793054255, -37.94852427682175744 ) ) ;
#10175=ORIENTED_EDGE ( 'NONE', *, *, #25212, .F. ) ;
#10188=FACE_BOUND ( 'NONE', #1456, .T. ) ;
#10251=EDGE_CURVE ( 'NONE', #23079, #13180, #19594, .T. ) ;
#10269=AXIS2_PLACEMENT_3D ( 'NONE', #30579, #18758, #2250 ) ;
#10270=ORIENTED_EDGE ( 'NONE', *, *, #25225, .F. ) ;
#10275=CYLINDRICAL_SURFACE ( 'NONE', #13019, 10.00000000000000533 ) ;
#10288=CARTESIAN_POINT ( 'NONE',  ( -7.999999999713793386, -30.00976070822369834, -28.70911656063094597 ) ) ;
#10300=ORIENTED_EDGE ( 'NONE', *, *, #20209, .F. ) ;
#10335=ORIENTED_EDGE ( 'NONE', *, *, #4405, .F. ) ;
#10336=FACE_OUTER_BOUND ( 'NONE', #1562, .T. ) ;
#10341=CARTESIAN_POINT ( 'NONE',  ( 8.700000000288207858, -19.62571037376041261, -40.87651877822478497 ) ) ;
#10344=EDGE_CURVE ( 'NONE', #16882, #6775, #14433, .T. ) ;
#10354=CARTESIAN_POINT ( 'NONE',  ( -8.699999999662093586, -15.94902145834643115, -35.53273252493492862 ) ) ;
#10410=CARTESIAN_POINT ( 'NONE',  ( 7.929582511818026092, -115.3684672989803630, 21.40105740852224159 ) ) ;
#10419=CARTESIAN_POINT ( 'NONE',  ( 8.700000000248305554, -25.92947359976189503, -31.20249410819006286 ) ) ;
#10421=CARTESIAN_POINT ( 'NONE',  ( 8.700000000248305554, -25.92947359976189503, -31.20249410819006286 ) ) ;
#10432=AXIS2_PLACEMENT_3D ( 'NONE', #2801, #7366, #9574 ) ;
#10441=ORIENTED_EDGE ( 'NONE', *, *, #30400, .F. ) ;
#10464=CARTESIAN_POINT ( 'NONE',  ( -7.999999999628359504, -14.95611408987656965, -40.37595097054163773 ) ) ;
#10467=EDGE_CURVE ( 'NONE', #5252, #3651, #26333, .T. ) ;
#10494=EDGE_LOOP ( 'NONE', ( #19908, #23815, #3942, #29074 ) ) ;
#10496=CARTESIAN_POINT ( 'NONE',  ( 8.000000000281882961, -22.83323352251018079, -39.84673050074155753 ) ) ;
#10503=CARTESIAN_POINT ( 'NONE',  ( 8.700000000270996736, -18.23122067931645773, -34.51216076560373125 ) ) ;
#10514=CARTESIAN_POINT ( 'NONE',  ( 8.700000000273361067, -18.09728189817007404, -34.21264730247137464 ) ) ;
#10526=EDGE_LOOP ( 'NONE', ( #2669, #20274, #15308, #17708, #8144, #23682, #16629, #20660 ) ) ;
#10539=CIRCLE ( 'NONE', #28127, 4.276011752367109509 ) ;
#10548=CLOSED_SHELL ( 'NONE', ( #30068, #6474, #371, #28541, #9891, #21421, #18484, #24036, #29673, #18128, #3284, #23948, #26632, #11529, #27790, #22620, #8255, #25460, #9559, #19833, #30796, #28487, #18915, #9327, #22918, #9143, #14247, #23266, #13454, #10820, #20664, #24112, #11737, #16128, #21622, #19009, #1575, #22860, #5418, #3428, #4328, #22025, #27322, #13118, #5444, #21959, #11040, #29435, #1404, #14989, #23433, #2967, #3967, #8930, #20726, #7683, #4668, #5357, #24928, #4442, #26348, #15412, #15200, #615, #8374, #6507, #27723, #8848, #7861 ) ) ;
#10559=LINE ( 'NONE', #29745, #30374 ) ;
#10573=CARTESIAN_POINT ( 'NONE',  ( -7.999999999652525950, -17.05009613497038146, -37.77893181949669099 ) ) ;
#10577=CARTESIAN_POINT ( 'NONE',  ( -7.439629836182230171, -5.610939228782946486, -27.11239056199590536 ) ) ;
#10608=VECTOR ( 'NONE', #1192, 1000.000000000000000 ) ;
#10617=DIRECTION ( 'NONE',  ( 2.764840495839172918E-12, 0.9128796883888953273, -0.4082287037029530552 ) ) ;
#10629=CARTESIAN_POINT ( 'NONE',  ( -7.999999999681657314, -14.84794678168725568, -33.28653323038288647 ) ) ;
#10645=ORIENTED_EDGE ( 'NONE', *, *, #3399, .F. ) ;
#10646=DIRECTION ( 'NONE',  ( -1.000000000000000000, 5.687697958343395332E-16, -6.771501495045879231E-12 ) ) ;
#10664=DIRECTION ( 'NONE',  ( 3.133604487004501912E-12, 0.3568421334038983650, -0.9341647027306021478 ) ) ;
#10696=LINE ( 'NONE', #657, #13137 ) ;
#10703=VERTEX_POINT ( 'NONE', #8663 ) ;
#10714=ORIENTED_EDGE ( 'NONE', *, *, #22431, .T. ) ;
#10723=CARTESIAN_POINT ( 'NONE',  ( -7.999999999674140660, -13.61361098168129224, -34.64062768038885309 ) ) ;
#10725=ORIENTED_EDGE ( 'NONE', *, *, #12332, .T. ) ;
#10731=CARTESIAN_POINT ( 'NONE',  ( -8.699999999701292452, -29.44961367803777463, -30.17582256626712223 ) ) ;
#10742=EDGE_LOOP ( 'NONE', ( #28366, #17483, #16127, #8172, #13228, #19657, #8485, #8565 ) ) ;
#10766=ORIENTED_EDGE ( 'NONE', *, *, #4472, .F. ) ;
#10790=AXIS2_PLACEMENT_3D ( 'NONE', #7333, #105, #9687 ) ;
#10797=EDGE_CURVE ( 'NONE', #28713, #8037, #3134, .T. ) ;
#10805=CARTESIAN_POINT ( 'NONE',  ( 8.700000000292124724, -17.59705092275675042, -40.94388382661216497 ) ) ;
#10820=ADVANCED_FACE ( 'NONE', ( #26911 ), #8152, .T. ) ;
#10849=CARTESIAN_POINT ( 'NONE',  ( -7.999999999938637529, -122.9973754718770493, 4.341317972039581363 ) ) ;
#10863=CYLINDRICAL_SURFACE ( 'NONE', #29367, 2.500000000000000888 ) ;
#10877=ORIENTED_EDGE ( 'NONE', *, *, #30437, .T. ) ;
#10899=DIRECTION ( 'NONE',  ( 3.084553072890618732E-12, 0.8902635789277789646, -0.4554456718805243165 ) ) ;
#10911=VERTEX_POINT ( 'NONE', #20591 ) ;
#10914=ORIENTED_EDGE ( 'NONE', *, *, #23516, .F. ) ;
#10928=FACE_BOUND ( 'NONE', #10526, .T. ) ;
#10932=ORIENTED_EDGE ( 'NONE', *, *, #15610, .T. ) ;
#10945=VECTOR ( 'NONE', #25784, 1000.000000000000000 ) ;
#10956=CARTESIAN_POINT ( 'NONE',  ( -8.699999999730072986, -28.07050130677435362, -25.59757157925566773 ) ) ;
#10960=ORIENTED_EDGE ( 'NONE', *, *, #7644, .T. ) ;
#10962=CARTESIAN_POINT ( 'NONE',  ( -4.276011752261355880, -43.23306002164930817, -10.18642677534438512 ) ) ;
#10976=CARTESIAN_POINT ( 'NONE',  ( -7.999999999720649235, -24.05737431392700287, -27.69631921959670251 ) ) ;
#10982=AXIS2_PLACEMENT_3D ( 'NONE', #8905, #23089, #4509 ) ;
#10984=FACE_OUTER_BOUND ( 'NONE', #11692, .T. ) ;
#10993=ORIENTED_EDGE ( 'NONE', *, *, #24054, .F. ) ;
#11003=AXIS2_PLACEMENT_3D ( 'NONE', #19637, #26714, #19486 ) ;
#11014=CARTESIAN_POINT ( 'NONE',  ( 8.000000000730963734, -26.52402217160887332, -25.41208138063096200 ) ) ;
#11032=ORIENTED_EDGE ( 'NONE', *, *, #11822, .T. ) ;
#11039=CARTESIAN_POINT ( 'NONE',  ( -8.699999998932284484, -16.96959321760381556, -37.81493174590716677 ) ) ;
#11040=ADVANCED_FACE ( 'NONE', ( #11620 ), #2184, .F. ) ;
#11041=ORIENTED_EDGE ( 'NONE', *, *, #12124, .T. ) ;
#11053=CARTESIAN_POINT ( 'NONE',  ( -8.699999999695858577, -28.58460556449822576, -30.97768745922355293 ) ) ;
#11070=CARTESIAN_POINT ( 'NONE',  ( 8.000000000235820252, -29.73863906515999389, -27.17531388883937993 ) ) ;
#11083=CARTESIAN_POINT ( 'NONE',  ( -7.999999999692728458, -26.29631921955218132, -31.34262568607297439 ) ) ;
#11093=LINE ( 'NONE', #18322, #4140 ) ;
#11097=B_SPLINE_CURVE_WITH_KNOTS ( 'NONE', 5,
 ( #11484, #30682, #16352, #3776, #25494, #6755, #4397, #14003, #9264, #18870, #22977, #11792 ),
 .UNSPECIFIED., .F., .F.,
 ( 6, 3, 3, 6 ),
 ( 11.50063931930000116, 13.17185654790000093, 19.75779804580000132, 23.00143448300000060 ),
 .UNSPECIFIED. ) ;
#11098=CARTESIAN_POINT ( 'NONE',  ( 8.000000000279957391, -18.28443193505134445, -36.42483736938841332 ) ) ;
#11110=CARTESIAN_POINT ( 'NONE',  ( 7.873274151039644231, -5.775076759590717757, -27.47943436997715594 ) ) ;
#11120=CARTESIAN_POINT ( 'NONE',  ( -8.699999999669890016, -18.36515956938880478, -34.81167447243381474 ) ) ;
#11123=CARTESIAN_POINT ( 'NONE',  ( -8.699999999662093586, -15.94902145834643115, -35.53273252493492862 ) ) ;
#11135=CARTESIAN_POINT ( 'NONE',  ( 8.700000000246973286, -27.86619909556666030, -31.29895010227025409 ) ) ;
#11154=CARTESIAN_POINT ( 'NONE',  ( -8.699999999945166707, -111.9817663798742444, 5.760339591697572814 ) ) ;
#11172=FACE_OUTER_BOUND ( 'NONE', #14025, .T. ) ;
#11192=CARTESIAN_POINT ( 'NONE',  ( 8.000000000278095769, -14.92844969908619035, -33.25053330389217621 ) ) ;
#11204=DIRECTION ( 'NONE',  ( 1.000000000000000000, -1.844929437980039379E-12, 2.650555428735150365E-12 ) ) ;
#11215=ORIENTED_EDGE ( 'NONE', *, *, #2619, .T. ) ;
#11253=CARTESIAN_POINT ( 'NONE',  ( 8.000000000248585152, -27.47644226431772907, -31.38783462175427630 ) ) ;
#11257=DIRECTION ( 'NONE',  ( -0.000000000000000000, 0.9128796883888952163, -0.4082287037029530552 ) ) ;
#11261=VECTOR ( 'NONE', #1081, 1000.000000000000000 ) ;
#11266=ORIENTED_EDGE ( 'NONE', *, *, #23823, .T. ) ;
#11273=ORIENTED_EDGE ( 'NONE', *, *, #29489, .F. ) ;
#11282=VECTOR ( 'NONE', #464, 999.9999999999998863 ) ;
#11285=DIRECTION ( 'NONE',  ( -6.326189572192214457E-12, -0.3568421334038989756, 0.9341647027306019258 ) ) ;
#11316=DIRECTION ( 'NONE',  ( 1.000000000000000000, -1.843431230200084908E-12, 2.650498504963248473E-12 ) ) ;
#11324=CARTESIAN_POINT ( 'NONE',  ( 8.000000000462277328, -18.10926874255784469, -36.88339488450507986 ) ) ;
#11384=ORIENTED_EDGE ( 'NONE', *, *, #9836, .T. ) ;
#11386=SURFACE_STYLE_FILL_AREA ( #15945 ) ;
#11432=DIRECTION ( 'NONE',  ( 1.000000000000000000, -1.843431230200084908E-12, 2.650498504963248473E-12 ) ) ;
#11436=DIRECTION ( 'NONE',  ( -1.000000000000000000, 5.687697913153403713E-16, -6.771501495041734442E-12 ) ) ;
#11446=CARTESIAN_POINT ( 'NONE',  ( -7.999999999717977595, -23.99023929173318948, -28.09088343939654209 ) ) ;
#11450=CARTESIAN_POINT ( 'NONE',  ( 8.700000000249984211, -26.29631921959126117, -31.34262568600063759 ) ) ;
#11456=AXIS2_PLACEMENT_3D ( 'NONE', #7077, #14329, #1480 ) ;
#11469=CARTESIAN_POINT ( 'NONE',  ( -8.699999999970339459, -115.7892272537997371, 9.034522706526081137 ) ) ;
#11479=CIRCLE ( 'NONE', #11003, 4.276011752367103291 ) ;
#11484=CARTESIAN_POINT ( 'NONE',  ( -7.999999999628359504, -14.95611408987656965, -40.37595097054163773 ) ) ;
#11487=CARTESIAN_POINT ( 'NONE',  ( 8.700000000289719537, -13.99335427294626832, -37.12410235030684902 ) ) ;
#11495=ORIENTED_EDGE ( 'NONE', *, *, #3659, .T. ) ;
#11513=EDGE_LOOP ( 'NONE', ( #23744, #831, #16675, #1754 ) ) ;
#11529=ADVANCED_FACE ( 'NONE', ( #13418 ), #28476, .F. ) ;
#11530=EDGE_LOOP ( 'NONE', ( #21155, #785, #23397, #24693 ) ) ;
#11537=VERTEX_POINT ( 'NONE', #11070 ) ;
#11540=( LENGTH_UNIT ( ) NAMED_UNIT ( * ) SI_UNIT ( .MILLI., .METRE. ) );
#11543=B_SPLINE_CURVE_WITH_KNOTS ( 'NONE', 5,
 ( #17226, #12358, #29181, #575, #26381, #24018, #10156, #19600, #2605, #29337, #21495, #5280 ),
 .UNSPECIFIED., .F., .F.,
 ( 6, 3, 3, 6 ),
 ( 2.782752057460000206, 3.293393370880000059, 4.940089941970000176, 5.565010780559999759 ),
 .UNSPECIFIED. ) ;
#11561=DIRECTION ( 'NONE',  ( -1.000000000000000000, 5.687697999151106851E-16, -6.771501495036750356E-12 ) ) ;
#11587=CARTESIAN_POINT ( 'NONE',  ( -8.699999999661049088, -18.40166527955781817, -36.11775795388252419 ) ) ;
#11620=FACE_OUTER_BOUND ( 'NONE', #27534, .T. ) ;
#11632=DIRECTION ( 'NONE',  ( 1.666951178525963134E-12, -0.4082287037029531107, -0.9128796883888953273 ) ) ;
#11641=DIRECTION ( 'NONE',  ( -1.000000000000000000, 5.687697937797165957E-16, -6.771501495045624776E-12 ) ) ;
#11646=CARTESIAN_POINT ( 'NONE',  ( 8.700000000246273402, -23.99025505878464060, -28.09032254495748049 ) ) ;
#11652=VERTEX_POINT ( 'NONE', #6111 ) ;
#11673=PLANE ( 'NONE',  #13114 ) ;
#11682=CARTESIAN_POINT ( 'NONE',  ( 8.700000000273695022, -16.20708930593283625, -33.02464488162291900 ) ) ;
#11692=EDGE_LOOP ( 'NONE', ( #12228, #10932, #2171, #18501 ) ) ;
#11702=ORIENTED_EDGE ( 'NONE', *, *, #10251, .F. ) ;
#11718=EDGE_CURVE ( 'NONE', #7680, #90, #13669, .T. ) ;
#11720=CARTESIAN_POINT ( 'NONE',  ( -7.999999999669004325, -18.23122067930106027, -34.51216076568240965 ) ) ;
#11737=ADVANCED_FACE ( 'NONE', ( #4382 ), #20915, .T. ) ;
#11742=DIRECTION ( 'NONE',  ( 1.000000000000000000, -9.219999999999999084E-13, 4.710999999999999616E-12 ) ) ;
#11759=CARTESIAN_POINT ( 'NONE',  ( 7.620434517626458515, -115.2052681231116509, 21.76600287036780301 ) ) ;
#11763=ORIENTED_EDGE ( 'NONE', *, *, #27821, .T. ) ;
#11769=VECTOR ( 'NONE', #22008, 1000.000000000000000 ) ;
#11775=CARTESIAN_POINT ( 'NONE',  ( -8.699999999649387306, -11.00382829991729849, -37.83919293449501708 ) ) ;
#11792=CARTESIAN_POINT ( 'NONE',  ( -7.999999999638116144, -22.83323352248630655, -39.84673050082100332 ) ) ;
#11812=ORIENTED_EDGE ( 'NONE', *, *, #18978, .T. ) ;
#11822=EDGE_CURVE ( 'NONE', #8842, #17525, #12966, .T. ) ;
#11826=ORIENTED_EDGE ( 'NONE', *, *, #30137, .T. ) ;
#11833=FACE_OUTER_BOUND ( 'NONE', #30058, .T. ) ;
#11840=CARTESIAN_POINT ( 'NONE',  ( 8.700000000270996736, -18.23122067931645773, -34.51216076560373125 ) ) ;
#11852=CARTESIAN_POINT ( 'NONE',  ( -7.999999999669917372, -18.13635916017433658, -34.30003174772016905 ) ) ;
#11859=ORIENTED_EDGE ( 'NONE', *, *, #30210, .F. ) ;
#11865=CARTESIAN_POINT ( 'NONE',  ( 8.000000000869471606, -28.58317312643325536, -30.97832802804627406 ) ) ;
#11920=CARTESIAN_POINT ( 'NONE',  ( -7.999999999650268201, -15.05691661382650537, -37.86814300153927348 ) ) ;
#11933=ORIENTED_EDGE ( 'NONE', *, *, #19427, .T. ) ;
#11949=AXIS2_PLACEMENT_3D ( 'NONE', #21646, #95, #24155 ) ;
#11953=CARTESIAN_POINT ( 'NONE',  ( -7.999999999654174410, -13.78556554857453698, -36.79016579852192592 ) ) ;
#11975=DIRECTION ( 'NONE',  ( -6.028162111955455897E-12, 0.4554456718800332649, 0.8902635789280302081 ) ) ;
#11986=EDGE_LOOP ( 'NONE', ( #16450, #24988, #13985, #7192 ) ) ;
#11991=VERTEX_POINT ( 'NONE', #27328 ) ;
#11996=CARTESIAN_POINT ( 'NONE',  ( 8.000000000264140709, -18.27877680372071723, -30.94409471150577318 ) ) ;
#12004=B_SPLINE_CURVE_WITH_KNOTS ( 'NONE', 3,
 ( #17863, #20398, #22296, #15366, #10341, #19934, #10805, #8419, #3556, #12688 ),
 .UNSPECIFIED., .F., .F.,
 ( 4, 2, 2, 2, 4 ),
 ( 0.000000000000000000, 0.2500000000000000000, 0.5000000000000000000, 0.7500000000000000000, 1.000000000000000000 ),
 .UNSPECIFIED. ) ;
#12007=LINE ( 'NONE', #2567, #2109 ) ;
#12032=FACE_OUTER_BOUND ( 'NONE', #24557, .T. ) ;
#12052=CARTESIAN_POINT ( 'NONE',  ( 8.700000000287184676, -13.53252229041972043, -36.25298318319556046 ) ) ;
#12082=EDGE_CURVE ( 'NONE', #2058, #19001, #9571, .T. ) ;
#12089=EDGE_CURVE ( 'NONE', #22839, #3906, #1440, .T. ) ;
#12098=CARTESIAN_POINT ( 'NONE',  ( 1.030019577584203890E-10, -106.6790623149837245, 18.95265870294618082 ) ) ;
#12111=VERTEX_POINT ( 'NONE', #1530 ) ;
#12112=CARTESIAN_POINT ( 'NONE',  ( -7.999999999730073696, -28.07052495761531219, -25.59750966829892960 ) ) ;
#12124=EDGE_CURVE ( 'NONE', #20972, #15836, #8441, .T. ) ;
#12128=CARTESIAN_POINT ( 'NONE',  ( -8.700000000050449600, -115.5267901941123370, 21.04701626955306537 ) ) ;
#12133=AXIS2_PLACEMENT_3D ( 'NONE', #30414, #9306, #11204 ) ;
#12138=CARTESIAN_POINT ( 'NONE',  ( -8.699999999674142614, -13.61360970150653316, -34.64062719139432289 ) ) ;
#12142=DIRECTION ( 'NONE',  ( -2.764840495839172918E-12, -0.9128796883888953273, 0.4082287037029531107 ) ) ;
#12152=ORIENTED_EDGE ( 'NONE', *, *, #7072, .T. ) ;
#12168=CARTESIAN_POINT ( 'NONE',  ( -8.699999998988344529, -24.19750589173278499, -27.32947359979484858 ) ) ;
#12177=CYLINDRICAL_SURFACE ( 'NONE', #26884, 3.000000000000002220 ) ;
#12181=ORIENTED_EDGE ( 'NONE', *, *, #23125, .F. ) ;
#12190=CARTESIAN_POINT ( 'NONE',  ( 8.700000000232341435, -25.77531388888509056, -25.66136093477824431 ) ) ;
#12195=PRODUCT_DEFINITION_CONTEXT ( 'detailed design', #4757, 'design' ) ;
#12214=CARTESIAN_POINT ( 'NONE',  ( -7.999999999730073696, -28.07052495761531219, -25.59750966829892960 ) ) ;
#12228=ORIENTED_EDGE ( 'NONE', *, *, #107, .T. ) ;
#12249=CARTESIAN_POINT ( 'NONE',  ( 4.276011752472853367, -9.320059656523383751, -25.35190844153497380 ) ) ;
#12265=ORIENTED_EDGE ( 'NONE', *, *, #12332, .F. ) ;
#12270=CARTESIAN_POINT ( 'NONE',  ( -7.999999999729050515, -26.29567537037302927, -25.46710523971266582 ) ) ;
#12276=CARTESIAN_POINT ( 'NONE',  ( 8.700000000285857737, -13.61366271048277277, -34.64064744186795508 ) ) ;
#12312=B_SPLINE_CURVE_WITH_KNOTS ( 'NONE', 3,
 ( #10956, #29984, #22921, #8417, #14947, #25442 ),
 .UNSPECIFIED., .F., .F.,
 ( 4, 2, 4 ),
 ( 0.000000000000000000, 0.5000000000000000000, 1.000000000000000000 ),
 .UNSPECIFIED. ) ;
#12332=EDGE_CURVE ( 'NONE', #23086, #7730, #28686, .T. ) ;
#12337=ORIENTED_EDGE ( 'NONE', *, *, #6445, .F. ) ;
#12358=CARTESIAN_POINT ( 'NONE',  ( -7.999999999683975460, -16.77380904890792834, -33.17160705600048942 ) ) ;
#12376=CARTESIAN_POINT ( 'NONE',  ( 7.999999999994048316, -116.8591659214849159, 11.34031266730467813 ) ) ;
#12395=CARTESIAN_POINT ( 'NONE',  ( 8.699999999949442397, -116.5561065468441626, 18.74526241745003574 ) ) ;
#12398=LINE ( 'NONE', #5620, #11282 ) ;
#12401=CARTESIAN_POINT ( 'NONE',  ( -8.699999999695283037, -25.56176843068484317, -31.06196806030030544 ) ) ;
#12407=CARTESIAN_POINT ( 'NONE',  ( 8.699999999957087837, -117.0726643325088645, 17.59013759100812280 ) ) ;
#12410=EDGE_LOOP ( 'NONE', ( #15168, #1628, #30676, #25343 ) ) ;
#12440=AXIS2_PLACEMENT_3D ( 'NONE', #9709, #445, #16786 ) ;
#12463=FACE_OUTER_BOUND ( 'NONE', #12533, .T. ) ;
#12478=DIRECTION ( 'NONE',  ( -1.000000000000000000, 5.687698019339887572E-16, -6.771501495046482653E-12 ) ) ;
#12493=ORIENTED_EDGE ( 'NONE', *, *, #6721, .T. ) ;
#12499=CIRCLE ( 'NONE', #28091, 10.00000000000000178 ) ;
#12502=CARTESIAN_POINT ( 'NONE',  ( 8.000000000875953532, -24.10104989775918938, -29.26619909572536926 ) ) ;
#12505=CARTESIAN_POINT ( 'NONE',  ( 8.700000000284758173, -13.44093381510830909, -35.27466467713743015 ) ) ;
#12525=ORIENTED_EDGE ( 'NONE', *, *, #12089, .F. ) ;
#12533=EDGE_LOOP ( 'NONE', ( #10960, #16986, #13501, #22571 ) ) ;
#12536=DIRECTION ( 'NONE',  ( 2.764840495839172514E-12, 0.9128796883888952163, -0.4082287037029530552 ) ) ;
#12551=EDGE_CURVE ( 'NONE', #2707, #27598, #15109, .T. ) ;
#12559=B_SPLINE_CURVE_WITH_KNOTS ( 'NONE', 5,
 ( #19401, #11852, #531, #23975, #5075, #7589, #21927, #7435, #2717 ),
 .UNSPECIFIED., .F., .F.,
 ( 6, 3, 6 ),
 ( 0.000000000000000000, 1.646696146380000059, 2.782752057460000206 ),
 .UNSPECIFIED. ) ;
#12604=CARTESIAN_POINT ( 'NONE',  ( 6.999999999942878581, -114.8328013981175673, 22.59891173924912877 ) ) ;
#12610=EDGE_LOOP ( 'NONE', ( #28821, #11826, #8780, #6025, #6143, #23972, #5344, #19319 ) ) ;
#12613=CARTESIAN_POINT ( 'NONE',  ( -7.999999999659028305, -18.20005812739434958, -36.62389201141883177 ) ) ;
#12630=CARTESIAN_POINT ( 'NONE',  ( -8.699999999628362346, -14.95623164695839513, -40.37561726986208299 ) ) ;
#12648=CIRCLE ( 'NONE', #30245, 1.699999999999999289 ) ;
#12649=ORIENTED_EDGE ( 'NONE', *, *, #19427, .F. ) ;
#12659=MECHANICAL_DESIGN_GEOMETRIC_PRESENTATION_REPRESENTATION('',(#23328),#5632);
#12688=CARTESIAN_POINT ( 'NONE',  ( 8.700000000301640668, -14.95611408989196711, -40.37595097046296644 ) ) ;
#12707=CARTESIAN_POINT ( 'NONE',  ( 8.700000000272996914, -17.90486156772228554, -33.94152562884548985 ) ) ;
#12718=EDGE_CURVE ( 'NONE', #19512, #30177, #18224, .T. ) ;
#12721=CARTESIAN_POINT ( 'NONE',  ( -8.699999999673119433, -13.73066623916353102, -34.33432129195676197 ) ) ;
#12736=CARTESIAN_POINT ( 'NONE',  ( 1.814857447021396585E-10, -114.8436363890427856, 0.6950649351682707255 ) ) ;
#12745=CARTESIAN_POINT ( 'NONE',  ( 8.000000000264140709, -18.27877680372071723, -30.94409471150577318 ) ) ;
#12770=EDGE_CURVE ( 'NONE', #19970, #725, #11479, .T. ) ;
#12780=CARTESIAN_POINT ( 'NONE',  ( 8.700000000244115128, -26.99999999999395328, -28.39999999994493862 ) ) ;
#12782=CARTESIAN_POINT ( 'NONE',  ( -7.572771919371899862, -5.645290041039670470, -27.18920573570797217 ) ) ;
#12796=B_SPLINE_CURVE_WITH_KNOTS ( 'NONE', 3,
 ( #13649, #11135, #23420, #23577, #11450, #22940 ),
 .UNSPECIFIED., .F., .F.,
 ( 4, 2, 4 ),
 ( 0.000000000000000000, 0.5000000000000000000, 1.000000000000000000 ),
 .UNSPECIFIED. ) ;
#12816=VERTEX_POINT ( 'NONE', #12395 ) ;
#12823=FACE_OUTER_BOUND ( 'NONE', #2306, .T. ) ;
#12838=VECTOR ( 'NONE', #28695, 999.9999999999998863 ) ;
#12908=CARTESIAN_POINT ( 'NONE',  ( -8.699999999724179034, -29.73863906514459643, -27.17531388891805477 ) ) ;
#12914=DIRECTION ( 'NONE',  ( 1.000000000000000000, -1.843431230200084908E-12, 2.650498504963248473E-12 ) ) ;
#12917=CARTESIAN_POINT ( 'NONE',  ( -7.999999999691694619, -25.92947359974649046, -31.20249410826873415 ) ) ;
#12920=ORIENTED_EDGE ( 'NONE', *, *, #16435, .F. ) ;
#12923=ORIENTED_EDGE ( 'NONE', *, *, #24895, .T. ) ;
#12928=CARTESIAN_POINT ( 'NONE',  ( -7.999999999654106908, -17.47950540273041753, -37.52766237889763801 ) ) ;
#12933=CARTESIAN_POINT ( 'NONE',  ( -7.195957063952547195, -5.577897551235623474, -27.03850287102680738 ) ) ;
#12936=AXIS2_PLACEMENT_3D ( 'NONE', #7052, #2641, #7515 ) ;
#12956=ORIENTED_EDGE ( 'NONE', *, *, #8289, .F. ) ;
#12958=AXIS2_PLACEMENT_3D ( 'NONE', #17668, #29950, #22418 ) ;
#12966=B_SPLINE_CURVE_WITH_KNOTS ( 'NONE', 3,
 ( #14141, #4073, #23746, #2183, #11775, #23907, #21381, #30972, #28613, #7051 ),
 .UNSPECIFIED., .F., .F.,
 ( 4, 2, 2, 2, 4 ),
 ( 0.000000000000000000, 0.2500000000000000000, 0.5000000000000000000, 0.7500000000000000000, 1.000000000000000000 ),
 .UNSPECIFIED. ) ;
#12974=DIRECTION ( 'NONE',  ( -1.000000000000000000, 5.687697999151106851E-16, -6.771501495036750356E-12 ) ) ;
#12984=DIRECTION ( 'NONE',  ( -7.759996349202911684E-13, -0.9341647027306021478, -0.3568421334038983650 ) ) ;
#13013=AXIS2_PLACEMENT_3D ( 'NONE', #28263, #4355, #11285 ) ;
#13019=AXIS2_PLACEMENT_3D ( 'NONE', #28688, #5386, #24592 ) ;
#13031=EDGE_LOOP ( 'NONE', ( #26677, #19276, #7608, #17656, #30695 ) ) ;
#13035=ORIENTED_EDGE ( 'NONE', *, *, #23125, .T. ) ;
#13054=CARTESIAN_POINT ( 'NONE',  ( -7.872160508897946052, -115.3203316365707849, 21.50869821882927724 ) ) ;
#13061=VECTOR ( 'NONE', #1899, 1000.000000000000000 ) ;
#13062=LINE ( 'NONE', #27537, #21813 ) ;
#13065=CYLINDRICAL_SURFACE ( 'NONE', #9289, 1.000000000000001332 ) ;
#13070=EDGE_LOOP ( 'NONE', ( #5865, #11041, #1834, #10766 ) ) ;
#13077=DIRECTION ( 'NONE',  ( 1.000000000000000000, -1.843431230198065828E-12, 2.650498504953516580E-12 ) ) ;
#13084=CARTESIAN_POINT ( 'NONE',  ( -8.699999999703575071, -29.66205794074117819, -29.83816939507471133 ) ) ;
#13089=VECTOR ( 'NONE', #13932, 1000.000000000000000 ) ;
#13114=AXIS2_PLACEMENT_3D ( 'NONE', #18438, #25693, #2081 ) ;
#13118=ADVANCED_FACE ( 'NONE', ( #4042 ), #1842, .F. ) ;
#13137=VECTOR ( 'NONE', #17616, 999.9999999999998863 ) ;
#13141=CARTESIAN_POINT ( 'NONE',  ( 7.973778855661143083, -5.874736698510242938, -27.70229359854242190 ) ) ;
#13147=EDGE_CURVE ( 'NONE', #8037, #14716, #30925, .T. ) ;
#13157=DIRECTION ( 'NONE',  ( -2.415891560877031462E-12, 0.9341647027306021478, 0.3568421334038983650 ) ) ;
#13161=CARTESIAN_POINT ( 'NONE',  ( -8.699999999707589637, -24.26136093481122558, -29.62468611113576955 ) ) ;
#13162=LINE ( 'NONE', #6404, #20796 ) ;
#13180=VERTEX_POINT ( 'NONE', #4513 ) ;
#13187=DIRECTION ( 'NONE',  ( 2.764840495839172918E-12, 0.9128796883888953273, -0.4082287037029530552 ) ) ;
#13193=CARTESIAN_POINT ( 'NONE',  ( -8.000000000040557779, -116.5561065465021784, 18.74526241810166027 ) ) ;
#13228=ORIENTED_EDGE ( 'NONE', *, *, #13252, .T. ) ;
#13250=DIRECTION ( 'NONE',  ( -2.416122857340496113E-12, 0.9341647027306024809, 0.3568421334038978099 ) ) ;
#13252=EDGE_CURVE ( 'NONE', #23341, #9577, #4658, .T. ) ;
#13262=AXIS2_PLACEMENT_3D ( 'NONE', #7831, #24984, #6091 ) ;
#13278=PLANE ( 'NONE',  #7944 ) ;
#13290=AXIS2_PLACEMENT_3D ( 'NONE', #2998, #15853, #18194 ) ;
#13306=FACE_OUTER_BOUND ( 'NONE', #6271, .T. ) ;
#13326=CARTESIAN_POINT ( 'NONE',  ( -8.699999999707452858, -24.10060434105348648, -29.26520274339392813 ) ) ;
#13369=EDGE_CURVE ( 'NONE', #2756, #20972, #12499, .T. ) ;
#13370=B_SPLINE_CURVE_WITH_KNOTS ( 'NONE', 5,
 ( #7378, #17277, #29087, #24527, #26578, #26887, #5326, #26725, #10056, #22166, #773, #19183, #624, #17124, #26429 ),
 .UNSPECIFIED., .F., .F.,
 ( 6, 3, 3, 3, 6 ),
 ( 10.75845894650000112, 13.17160129120000001, 18.65982206369999830, 20.85462967400000167, 21.51695457350000140 ),
 .UNSPECIFIED. ) ;
#13373=FACE_OUTER_BOUND ( 'NONE', #6574, .T. ) ;
#13376=DIRECTION ( 'NONE',  ( -1.000000000000000000, 2.082932338114093583E-15, -6.768115529734696084E-12 ) ) ;
#13378=EDGE_LOOP ( 'NONE', ( #7870, #17324, #173, #23268 ) ) ;
#13389=CARTESIAN_POINT ( 'NONE',  ( 8.699999999559956620, -18.28443321520602183, -36.42483785839191768 ) ) ;
#13418=FACE_OUTER_BOUND ( 'NONE', #16334, .T. ) ;
#13420=ORIENTED_EDGE ( 'NONE', *, *, #27315, .F. ) ;
#13425=CARTESIAN_POINT ( 'NONE',  ( -8.699999999669005391, -18.23122067931867107, -34.51216076567753532 ) ) ;
#13429=B_SPLINE_CURVE_WITH_KNOTS ( 'NONE', 3,
 ( #1, #1738, #9422, #6446, #9113, #16509 ),
 .UNSPECIFIED., .F., .F.,
 ( 4, 2, 4 ),
 ( 0.000000000000000000, 0.5000000000000000000, 1.000000000000000000 ),
 .UNSPECIFIED. ) ;
#13451=FACE_OUTER_BOUND ( 'NONE', #11986, .T. ) ;
#13454=ADVANCED_FACE ( 'NONE', ( #6044 ), #22268, .F. ) ;
#13478=EDGE_LOOP ( 'NONE', ( #8378, #5059, #30209, #6157 ) ) ;
#13486=EDGE_CURVE ( 'NONE', #21601, #23040, #20067, .T. ) ;
#13498=ORIENTED_EDGE ( 'NONE', *, *, #29496, .F. ) ;
#13501=ORIENTED_EDGE ( 'NONE', *, *, #24895, .F. ) ;
#13506=EDGE_CURVE ( 'NONE', #17663, #11652, #3685, .T. ) ;
#13508=SURFACE_STYLE_FILL_AREA ( #27825 ) ;
#13529=B_SPLINE_CURVE_WITH_KNOTS ( 'NONE', 5,
 ( #16827, #24804, #7078, #21712, #19353, #16666, #19508, #21409, #11953, #26435, #14331, #2214 ),
 .UNSPECIFIED., .F., .F.,
 ( 6, 3, 3, 6 ),
 ( 2.782752056640000138, 3.293393369919999980, 4.940089939659999985, 5.565010778129999558 ),
 .UNSPECIFIED. ) ;
#13532=CARTESIAN_POINT ( 'NONE',  ( 8.700000000287717583, -16.96959321760160222, -37.81493174583334849 ) ) ;
#13564=B_SPLINE_CURVE_WITH_KNOTS ( 'NONE', 3,
 ( #2615, #16927, #29043, #24027, #273, #19919 ),
 .UNSPECIFIED., .F., .F.,
 ( 4, 2, 4 ),
 ( 0.000000000000000000, 0.5000000000000000000, 1.000000000000000000 ),
 .UNSPECIFIED. ) ;
#13567=CARTESIAN_POINT ( 'NONE',  ( -7.614137047376521750, -115.2001938015495028, 21.77735005150014302 ) ) ;
#13572=LINE ( 'NONE', #6799, #21833 ) ;
#13639=CARTESIAN_POINT ( 'NONE',  ( 8.700000000245887932, -28.22468611110281245, -31.13863906511161517 ) ) ;
#13649=CARTESIAN_POINT ( 'NONE',  ( 8.700000000245887932, -28.22468611110281245, -31.13863906511161517 ) ) ;
#13652=B_SPLINE_CURVE_WITH_KNOTS ( 'NONE', 3,
 ( #13161, #13326, #24974, #1538, #22768, #30491 ),
 .UNSPECIFIED., .F., .F.,
 ( 4, 2, 4 ),
 ( 0.000000000000000000, 0.5000000000000000000, 1.000000000000000000 ),
 .UNSPECIFIED. ) ;
#13665=VERTEX_POINT ( 'NONE', #29304 ) ;
#13669=LINE ( 'NONE', #16641, #26546 ) ;
#13684=CARTESIAN_POINT ( 'NONE',  ( -7.999999999703424791, -29.80249410822368006, -29.47052640025566816 ) ) ;
#13705=LINE ( 'NONE', #11039, #14475 ) ;
#13715=EDGE_LOOP ( 'NONE', ( #15128, #24194, #25145, #4616 ) ) ;
#13726=EDGE_CURVE ( 'NONE', #19159, #8911, #5708, .T. ) ;
#13727=ORIENTED_EDGE ( 'NONE', *, *, #13147, .F. ) ;
#13733=CARTESIAN_POINT ( 'NONE',  ( 8.700000000274950906, -15.55224769787477257, -33.04262248272473812 ) ) ;
#13740=ORIENTED_EDGE ( 'NONE', *, *, #13800, .F. ) ;
#13747=CIRCLE ( 'NONE', #13262, 1.700000000000000178 ) ;
#13750=CARTESIAN_POINT ( 'NONE',  ( 8.000000000485913532, -30.00976070830145304, -28.70911655965779730 ) ) ;
#13781=ORIENTED_EDGE ( 'NONE', *, *, #421, .F. ) ;
#13800=EDGE_CURVE ( 'NONE', #725, #6775, #24908, .T. ) ;
#13811=DIRECTION ( 'NONE',  ( -3.927995826131583318E-12, 0.4082287037029531107, 0.9128796883888953273 ) ) ;
#13814=AXIS2_PLACEMENT_3D ( 'NONE', #3654, #1311, #13250 ) ;
#13815=DIRECTION ( 'NONE',  ( -1.000000000000000000, 5.687698019339887572E-16, -6.771501495046482653E-12 ) ) ;
#13826=VECTOR ( 'NONE', #13832, 1000.000000000000000 ) ;
#13832=DIRECTION ( 'NONE',  ( -1.000000000000000000, 5.687697999151106851E-16, -6.771501495036750356E-12 ) ) ;
#13844=DIRECTION ( 'NONE',  ( 1.000000000000000000, -9.219545062029677348E-13, 4.710284450064082408E-12 ) ) ;
#13869=DIRECTION ( 'NONE',  ( -1.000000000000000000, 5.687697999151106851E-16, -6.771501495036750356E-12 ) ) ;
#13888=VERTEX_POINT ( 'NONE', #5698 ) ;
#13898=EDGE_CURVE ( 'NONE', #8911, #29654, #1197, .T. ) ;
#13899=CARTESIAN_POINT ( 'NONE',  ( -6.999999999595749145, -114.9756814440741124, 22.27940384897737403 ) ) ;
#13904=ORIENTED_EDGE ( 'NONE', *, *, #402, .T. ) ;
#13929=PLANE ( 'NONE',  #20287 ) ;
#13932=DIRECTION ( 'NONE',  ( 1.000000000000000000, -1.843431230200084908E-12, 2.650498504963248473E-12 ) ) ;
#13934=PRODUCT ( 'Moving Handle', 'Moving Handle', '', ( #23269 ) ) ;
#13936=LINE ( 'NONE', #20703, #18270 ) ;
#13939=ORIENTED_EDGE ( 'NONE', *, *, #19458, .F. ) ;
#13956=EDGE_CURVE ( 'NONE', #14873, #10703, #8673, .T. ) ;
#13960=CARTESIAN_POINT ( 'NONE',  ( 4.276011752548591005, -51.11187400310260642, -27.80500476121942199 ) ) ;
#13963=DIRECTION ( 'NONE',  ( 3.084561942502618954E-12, 0.8902635789277789646, -0.4554456718805243165 ) ) ;
#13974=LINE ( 'NONE', #26243, #10945 ) ;
#13985=ORIENTED_EDGE ( 'NONE', *, *, #23388, .T. ) ;
#13990=B_SPLINE_CURVE_WITH_KNOTS ( 'NONE', 3,
 ( #6479, #13567, #28191, #6329, #9305, #28349 ),
 .UNSPECIFIED., .F., .F.,
 ( 4, 2, 4 ),
 ( 0.000000000000000000, 0.5000000000000000000, 1.000000000000000000 ),
 .UNSPECIFIED. ) ;
#13991=LINE ( 'NONE', #23276, #13826 ) ;
#14001=CARTESIAN_POINT ( 'NONE',  ( -7.999999999826271413, -29.66236253007011925, -29.83737202115235121 ) ) ;
#14003=CARTESIAN_POINT ( 'NONE',  ( -7.999999999631178582, -20.24958040245157420, -40.81349356744964751 ) ) ;
#14013=CARTESIAN_POINT ( 'NONE',  ( 8.700000000241654874, -24.19757157926353486, -27.32949869323976699 ) ) ;
#14015=DIRECTION ( 'NONE',  ( 0.000000000000000000, 0.000000000000000000, 1.000000000000000000 ) ) ;
#14025=EDGE_LOOP ( 'NONE', ( #13035, #1675, #23904, #25263 ) ) ;
#14051=ORIENTED_EDGE ( 'NONE', *, *, #29648, .T. ) ;
#14073=EDGE_CURVE ( 'NONE', #16100, #21330, #19338, .T. ) ;
#14082=CARTESIAN_POINT ( 'NONE',  ( -8.699999999684717267, -16.53542210648553024, -33.08054445275527655 ) ) ;
#14087=FACE_OUTER_BOUND ( 'NONE', #16090, .T. ) ;
#14090=CARTESIAN_POINT ( 'NONE',  ( -7.999999999662342987, -18.41955439558022078, -35.96306069475997447 ) ) ;
#14092=EDGE_CURVE ( 'NONE', #11652, #30584, #18057, .T. ) ;
#14104=EDGE_LOOP ( 'NONE', ( #30543, #22266, #21645, #8523 ) ) ;
#14107=CARTESIAN_POINT ( 'NONE',  ( -8.699999999667697992, -18.43894776734996910, -35.13584674166673949 ) ) ;
#14113=CARTESIAN_POINT ( 'NONE',  ( -7.707106781243226123, -115.2381289094444128, 21.69251968763726879 ) ) ;
#14123=CARTESIAN_POINT ( 'NONE',  ( -7.999999999727738675, -29.19518467809294293, -26.31283570863942245 ) ) ;
#14136=B_SPLINE_CURVE_WITH_KNOTS ( 'NONE', 5,
 ( #9652, #14692, #19254, #7298, #24136, #14854, #18939, #16886, #24282 ),
 .UNSPECIFIED., .F., .F.,
 ( 6, 3, 6 ),
 ( 0.000000000000000000, 1.646696146280000050, 2.782752056640000138 ),
 .UNSPECIFIED. ) ;
#14141=CARTESIAN_POINT ( 'NONE',  ( -8.699999999668209583, -9.149979920083866958, -35.02638174926116221 ) ) ;
#14143=CIRCLE ( 'NONE', #14665, 1.700000000000000178 ) ;
#14146=DIRECTION ( 'NONE',  ( 2.764840495839172918E-12, 0.9128796883888953273, -0.4082287037029531107 ) ) ;
#14181=CARTESIAN_POINT ( 'NONE',  ( 8.700000000277558598, -14.62893623595633485, -33.38447208503446006 ) ) ;
#14213=CARTESIAN_POINT ( 'NONE',  ( 7.999999999977091214, -107.4273096626279482, 14.66297538114749344 ) ) ;
#14216=CARTESIAN_POINT ( 'NONE',  ( 1.814857447021396585E-10, -51.11187400310945605, -27.80500476123474485 ) ) ;
#14223=ORIENTED_EDGE ( 'NONE', *, *, #9967, .F. ) ;
#14232=LINE ( 'NONE', #12168, #27844 ) ;
#14247=ADVANCED_FACE ( 'NONE', ( #8437, #15684, #22774 ), #1542, .T. ) ;
#14263=CARTESIAN_POINT ( 'NONE',  ( 8.700000000296432390, -13.70519490899241788, -39.86245227785762779 ) ) ;
#14271=AXIS2_PLACEMENT_3D ( 'NONE', #2049, #23765, #7070 ) ;
#14276=LINE ( 'NONE', #23879, #25072 ) ;
#14286=DIRECTION ( 'NONE',  ( 1.000000000000000000, -1.843431230200084908E-12, 2.650498504963248473E-12 ) ) ;
#14287=ORIENTED_EDGE ( 'NONE', *, *, #7317, .F. ) ;
#14296=CARTESIAN_POINT ( 'NONE',  ( 8.700000000232341435, -25.77531388888509056, -25.66136093477824431 ) ) ;
#14317=B_SPLINE_CURVE_WITH_KNOTS ( 'NONE', 3,
 ( #30378, #4557, #23293, #11487, #28312, #30685 ),
 .UNSPECIFIED., .F., .F.,
 ( 4, 2, 4 ),
 ( 0.000000000000000000, 0.5000000000000000000, 1.000000000000000000 ),
 .UNSPECIFIED. ) ;
#14323=CARTESIAN_POINT ( 'NONE',  ( 8.700000000277906764, -15.94902145836247342, -35.53273252485295330 ) ) ;
#14324=CARTESIAN_POINT ( 'NONE',  ( 8.000000000270995670, -18.23122067931581114, -34.51216076560703527 ) ) ;
#14329=DIRECTION ( 'NONE',  ( 1.000000000000000000, -1.843431230208684274E-12, 2.650498504958264790E-12 ) ) ;
#14331=CARTESIAN_POINT ( 'NONE',  ( -7.999999999654833438, -13.70282216375966300, -36.63380720155397086 ) ) ;
#14346=CARTESIAN_POINT ( 'NONE',  ( 8.700000000281731261, -13.73096375760723653, -34.33359398852594069 ) ) ;
#14354=PLANE ( 'NONE',  #7258 ) ;
#14378=FACE_OUTER_BOUND ( 'NONE', #26286, .T. ) ;
#14413=CARTESIAN_POINT ( 'NONE',  ( 1.030019577584204020E-10, -42.94729992905040206, -9.547410993456834305 ) ) ;
#14419=DIRECTION ( 'NONE',  ( -1.000000000000000000, -1.091125017015992317E-13, -6.718390282834052461E-12 ) ) ;
#14433=CIRCLE ( 'NONE', #28999, 4.276011752367102403 ) ;
#14441=ORIENTED_EDGE ( 'NONE', *, *, #2908, .T. ) ;
#14444=EDGE_CURVE ( 'NONE', #3666, #23754, #14276, .T. ) ;
#14475=VECTOR ( 'NONE', #8818, 1000.000000000000000 ) ;
#14486=EDGE_CURVE ( 'NONE', #4237, #15963, #13564, .T. ) ;
#14490=CARTESIAN_POINT ( 'NONE',  ( 8.700000000277906764, -15.94902145836247342, -35.53273252485295330 ) ) ;
#14491=ORIENTED_EDGE ( 'NONE', *, *, #22912, .T. ) ;
#14532=ORIENTED_EDGE ( 'NONE', *, *, #23823, .F. ) ;
#14558=B_SPLINE_CURVE_WITH_KNOTS ( 'NONE', 4,
 ( #945, #29254, #17299, #26907, #17601 ),
 .UNSPECIFIED., .F., .F.,
 ( 5, 5 ),
 ( -0.9817477042459999970, 0.9817477042459999970 ),
 .UNSPECIFIED. ) ;
#14571=VECTOR ( 'NONE', #1289, 1000.000000000000000 ) ;
#14578=CARTESIAN_POINT ( 'NONE',  ( 8.700000000295537106, -10.55542841719123537, -37.33290089570849801 ) ) ;
#14586=CARTESIAN_POINT ( 'NONE',  ( -8.699999999724179034, -29.73863906514459643, -27.17531388891805477 ) ) ;
#14589=CARTESIAN_POINT ( 'NONE',  ( 8.000000000229924524, -28.07052495763006661, -25.59750966822355522 ) ) ;
#14601=CYLINDRICAL_SURFACE ( 'NONE', #12440, 4.276011752367109509 ) ;
#14607=EDGE_CURVE ( 'NONE', #3906, #10703, #15037, .T. ) ;
#14634=ORIENTED_EDGE ( 'NONE', *, *, #26690, .F. ) ;
#14635=EDGE_CURVE ( 'NONE', #24995, #61, #9510, .T. ) ;
#14644=CARTESIAN_POINT ( 'NONE',  ( -7.999999999730130540, -27.01023037466701737, -25.37764016532643652 ) ) ;
#14650=EDGE_CURVE ( 'NONE', #13665, #28711, #17999, .T. ) ;
#14665=AXIS2_PLACEMENT_3D ( 'NONE', #4244, #6442, #13844 ) ;
#14674=DIRECTION ( 'NONE',  ( -2.764840495839172918E-12, -0.9128796883888953273, 0.4082287037029530552 ) ) ;
#14679=EDGE_LOOP ( 'NONE', ( #25543, #11933, #5866, #30912 ) ) ;
#14683=CARTESIAN_POINT ( 'NONE',  ( -7.974324478553856288, -5.875456860424912442, -27.70390402236215976 ) ) ;
#14692=CARTESIAN_POINT ( 'NONE',  ( -7.999999999651639548, -16.75746419958745648, -37.90979326505508595 ) ) ;
#14706=VECTOR ( 'NONE', #2542, 1000.000000000000000 ) ;
#14708=CARTESIAN_POINT ( 'NONE',  ( 8.700000000244115128, -26.99999999999395328, -28.39999999994493862 ) ) ;
#14716=VERTEX_POINT ( 'NONE', #8720 ) ;
#14720=CARTESIAN_POINT ( 'NONE',  ( 8.700000000241654874, -24.19757157926353486, -27.32949869323976699 ) ) ;
#14725=CARTESIAN_POINT ( 'NONE',  ( 8.700000000283790058, -13.49664205606710787, -34.94696692446570552 ) ) ;
#14769=CARTESIAN_POINT ( 'NONE',  ( -8.699999999702578535, -24.42241997903665407, -29.98484581762153667 ) ) ;
#14779=AXIS2_PLACEMENT_3D ( 'NONE', #4669, #19303, #16931 ) ;
#14812=DIRECTION ( 'NONE',  ( 6.326189572192215265E-12, 0.3568421334038983650, -0.9341647027306021478 ) ) ;
#14831=CARTESIAN_POINT ( 'NONE',  ( 7.867249199797543113, -115.3182685132986904, 21.51331176843062210 ) ) ;
#14832=VECTOR ( 'NONE', #13811, 999.9999999999998863 ) ;
#14843=CARTESIAN_POINT ( 'NONE',  ( 8.000000000111514353, -60.34578018690848467, -2.533826264238200121 ) ) ;
#14847=CARTESIAN_POINT ( 'NONE',  ( -7.999999999674140660, -13.61361098168129224, -34.64062768038885309 ) ) ;
#14854=CARTESIAN_POINT ( 'NONE',  ( -7.999999999650055926, -15.51869328868451170, -38.00326546224398783 ) ) ;
#14870=ORIENTED_EDGE ( 'NONE', *, *, #1903, .T. ) ;
#14873=VERTEX_POINT ( 'NONE', #18946 ) ;
#14888=LINE ( 'NONE', #8089, #16194 ) ;
#14889=DIRECTION ( 'NONE',  ( -7.759996349202911684E-13, -0.9341647027306021478, -0.3568421334038983650 ) ) ;
#14909=EDGE_CURVE ( 'NONE', #6775, #17179, #233, .T. ) ;
#14926=CARTESIAN_POINT ( 'NONE',  ( -8.699999999707589637, -24.26136093481122558, -29.62468611113576955 ) ) ;
#14936=ORIENTED_EDGE ( 'NONE', *, *, #12718, .F. ) ;
#14938=ORIENTED_EDGE ( 'NONE', *, *, #25123, .T. ) ;
#14945=ORIENTED_EDGE ( 'NONE', *, *, #27192, .F. ) ;
#14947=CARTESIAN_POINT ( 'NONE',  ( -8.699999999730728462, -26.13380090399637368, -25.50104989788441756 ) ) ;
#14948=B_SPLINE_CURVE_WITH_KNOTS ( 'NONE', 3,
 ( #236, #24607, #17054, #10288, #19890, #29471 ),
 .UNSPECIFIED., .F., .F.,
 ( 4, 2, 4 ),
 ( 0.000000000000000000, 0.5000000000000000000, 1.000000000000000000 ),
 .UNSPECIFIED. ) ;
#14967=CARTESIAN_POINT ( 'NONE',  ( -8.699999999730072986, -28.07050130677435362, -25.59757157925566773 ) ) ;
#14968=EDGE_CURVE ( 'NONE', #17625, #15429, #7859, .T. ) ;
#14989=ADVANCED_FACE ( 'NONE', ( #9658 ), #17197, .F. ) ;
#15000=CARTESIAN_POINT ( 'NONE',  ( -4.276011752185619130, -51.11187400311629858, -27.80500476125005704 ) ) ;
#15001=LINE ( 'NONE', #24447, #28256 ) ;
#15023=CARTESIAN_POINT ( 'NONE',  ( -7.999999999994412470, -117.3221216070908355, 13.04594386772275527 ) ) ;
#15029=EDGE_CURVE ( 'NONE', #28198, #19001, #4797, .T. ) ;
#15037=CIRCLE ( 'NONE', #1477, 10.00000000000000355 ) ;
#15109=LINE ( 'NONE', #17003, #25040 ) ;
#15128=ORIENTED_EDGE ( 'NONE', *, *, #6995, .F. ) ;
#15161=VERTEX_POINT ( 'NONE', #31011 ) ;
#15168=ORIENTED_EDGE ( 'NONE', *, *, #713, .T. ) ;
#15186=DIRECTION ( 'NONE',  ( 0.000000000000000000, -0.9128796883888953273, 0.4082287037029528332 ) ) ;
#15200=ADVANCED_FACE ( 'NONE', ( #2529 ), #19366, .F. ) ;
#15214=CARTESIAN_POINT ( 'NONE',  ( 8.700000000284079604, -17.26910668097993096, -37.68099296457697278 ) ) ;
#15231=CARTESIAN_POINT ( 'NONE',  ( -8.699999998953916958, -16.84112679184576677, -33.19732076807623145 ) ) ;
#15244=VERTEX_POINT ( 'NONE', #9920 ) ;
#15261=AXIS2_PLACEMENT_3D ( 'NONE', #27641, #28119, #25617 ) ;
#15268=VECTOR ( 'NONE', #20125, 999.9999999999998863 ) ;
#15275=CARTESIAN_POINT ( 'NONE',  ( -7.999999999723122812, -24.55065533306149916, -26.62378963206735349 ) ) ;
#15278=DIRECTION ( 'NONE',  ( 2.848302087110504847E-12, 0.8902635789277789646, -0.4554456718805243165 ) ) ;
#15287=CARTESIAN_POINT ( 'NONE',  ( 8.700000000248291343, -24.65319937758141222, -30.30964379061154190 ) ) ;
#15308=ORIENTED_EDGE ( 'NONE', *, *, #27518, .T. ) ;
#15316=CARTESIAN_POINT ( 'NONE',  ( -8.699999999669005391, -18.23122067931867107, -34.51216076567753532 ) ) ;
#15351=ORIENTED_EDGE ( 'NONE', *, *, #27315, .T. ) ;
#15362=DIRECTION ( 'NONE',  ( 0.7071067811898220645, -0.2886612846638017538, -0.6455034180634621199 ) ) ;
#15366=CARTESIAN_POINT ( 'NONE',  ( 8.700000000286674862, -20.29216153631914210, -40.76320817051012568 ) ) ;
#15372=DIRECTION ( 'NONE',  ( 1.000000000000000000, -1.953112501701599149E-12, 2.703609717165946368E-12 ) ) ;
#15412=ADVANCED_FACE ( 'NONE', ( #23051, #10928, #17985 ), #13278, .T. ) ;
#15421=CARTESIAN_POINT ( 'NONE',  ( 8.000000000733132666, -29.34680062213522689, -26.49035620890133202 ) ) ;
#15425=VECTOR ( 'NONE', #30936, 999.9999999999998863 ) ;
#15429=VERTEX_POINT ( 'NONE', #22726 ) ;
#15435=CARTESIAN_POINT ( 'NONE',  ( -5.797918472035167525, -115.0360660101943182, 22.14437208026542692 ) ) ;
#15447=AXIS2_PLACEMENT_3D ( 'NONE', #10849, #8007, #950 ) ;
#15454=AXIS2_PLACEMENT_3D ( 'NONE', #3562, #5770, #13157 ) ;
#15462=ORIENTED_EDGE ( 'NONE', *, *, #20299, .F. ) ;
#15476=VECTOR ( 'NONE', #6816, 1000.000000000000000 ) ;
#15480=AXIS2_PLACEMENT_3D ( 'NONE', #26349, #12478, #7147 ) ;
#15557=CARTESIAN_POINT ( 'NONE',  ( 8.000000000836360314, -17.41770198678077719, -37.61454294949587052 ) ) ;
#15579=DIRECTION ( 'NONE',  ( 0.7071067811842725037, 0.2886612846624971307, 0.6455034180701249014 ) ) ;
#15591=LINE ( 'NONE', #25196, #14571 ) ;
#15594=B_SPLINE_CURVE_WITH_KNOTS ( 'NONE', 3,
 ( #23721, #21355, #7030, #30951, #16466, #26227 ),
 .UNSPECIFIED., .F., .F.,
 ( 4, 2, 4 ),
 ( 0.000000000000000000, 0.5000000000000000000, 1.000000000000000000 ),
 .UNSPECIFIED. ) ;
#15610=EDGE_CURVE ( 'NONE', #17625, #29694, #21771, .T. ) ;
#15629=CARTESIAN_POINT ( 'NONE',  ( -8.699999999629596914, -20.29243514309546370, -40.76306209186606822 ) ) ;
#15634=EDGE_CURVE ( 'NONE', #9121, #13665, #9761, .T. ) ;
#15648=CARTESIAN_POINT ( 'NONE',  ( 8.000000000832923064, -18.43160947565852226, -34.96026953474216725 ) ) ;
#15683=DIRECTION ( 'NONE',  ( 2.764840495839172918E-12, 0.9128796883888953273, -0.4082287037029531107 ) ) ;
#15684=FACE_BOUND ( 'NONE', #29644, .T. ) ;
#15719=DIRECTION ( 'NONE',  ( -7.764622278472185525E-13, -0.9341647027306024809, -0.3568421334038978099 ) ) ;
#15741=ORIENTED_EDGE ( 'NONE', *, *, #24537, .T. ) ;
#15772=ORIENTED_EDGE ( 'NONE', *, *, #20209, .T. ) ;
#15807=B_SPLINE_CURVE_WITH_KNOTS ( 'NONE', 3,
 ( #15316, #24457, #555, #26967, #3194, #22406 ),
 .UNSPECIFIED., .F., .F.,
 ( 4, 2, 4 ),
 ( 0.000000000000000000, 0.5000000000000000000, 1.000000000000000000 ),
 .UNSPECIFIED. ) ;
#15814=DIRECTION ( 'NONE',  ( -3.924189347185962345E-12, 0.4082287037029531107, 0.9128796883888953273 ) ) ;
#15836=VERTEX_POINT ( 'NONE', #26261 ) ;
#15843=LINE ( 'NONE', #25605, #8005 ) ;
#15853=DIRECTION ( 'NONE',  ( 2.764840495839172918E-12, 0.9128796883888953273, -0.4082287037029531107 ) ) ;
#15854=CARTESIAN_POINT ( 'NONE',  ( 8.700000000284820345, -13.66682223737197610, -36.55330428411850363 ) ) ;
#15857=CARTESIAN_POINT ( 'NONE',  ( -7.707106507371444870, -5.692566414263196428, -27.29492500646317765 ) ) ;
#15876=CARTESIAN_POINT ( 'NONE',  ( 8.000000000115440102, -60.75400889061143772, -3.446705952627092895 ) ) ;
#15895=CARTESIAN_POINT ( 'NONE',  ( 8.000000000859367688, -29.57832802809286932, -26.81682687350731342 ) ) ;
#15896=CARTESIAN_POINT ( 'NONE',  ( 8.700000000236576270, -29.80249410823907752, -29.47052640017699687 ) ) ;
#15907=ORIENTED_EDGE ( 'NONE', *, *, #29880, .T. ) ;
#15932=VERTEX_POINT ( 'NONE', #27478 ) ;
#15943=EDGE_LOOP ( 'NONE', ( #23707, #3484, #25398, #11273 ) ) ;
#15945=FILL_AREA_STYLE ('',( #6348 ) ) ;
#15963=VERTEX_POINT ( 'NONE', #8279 ) ;
#15964=DIRECTION ( 'NONE',  ( -1.000000000000000000, 5.687697999151106851E-16, -6.771501495036750356E-12 ) ) ;
#15988=VERTEX_POINT ( 'NONE', #16002 ) ;
#16002=CARTESIAN_POINT ( 'NONE',  ( 8.700000000289733748, -15.05693637256081097, -37.86809127166881694 ) ) ;
#16005=FACE_OUTER_BOUND ( 'NONE', #27982, .T. ) ;
#16018=VECTOR ( 'NONE', #17504, 1000.000000000000114 ) ;
#16028=VECTOR ( 'NONE', #26220, 999.9999999999998863 ) ;
#16030=DIRECTION ( 'NONE',  ( -3.924189347185961537E-12, 0.4082287037029530552, 0.9128796883888952163 ) ) ;
#16074=CARTESIAN_POINT ( 'NONE',  ( -7.999999999671841167, -13.47848852103334671, -35.10240435524886493 ) ) ;
#16090=EDGE_LOOP ( 'NONE', ( #25909, #14532, #29037, #24726 ) ) ;
#16096=CARTESIAN_POINT ( 'NONE',  ( -8.699999999707589637, -24.26136093481122558, -29.62468611113576955 ) ) ;
#16100=VERTEX_POINT ( 'NONE', #14113 ) ;
#16127=ORIENTED_EDGE ( 'NONE', *, *, #4472, .T. ) ;
#16128=ADVANCED_FACE ( 'NONE', ( #30947 ), #4971, .T. ) ;
#16129=CARTESIAN_POINT ( 'NONE',  ( -8.699999999988495603, -117.2796036019060466, 12.53378552382356403 ) ) ;
#16161=DIRECTION ( 'NONE',  ( 1.000000000000000000, -1.843431230206220100E-12, 2.650498504954374861E-12 ) ) ;
#16171=EDGE_CURVE ( 'NONE', #9577, #12816, #14888, .T. ) ;
#16177=ORIENTED_EDGE ( 'NONE', *, *, #18821, .T. ) ;
#16185=CARTESIAN_POINT ( 'NONE',  ( 8.000000000468180161, -13.43844522892069371, -35.09918421751434892 ) ) ;
#16194=VECTOR ( 'NONE', #17538, 999.9999999999998863 ) ;
#16209=AXIS2_PLACEMENT_3D ( 'NONE', #8261, #30303, #3869 ) ;
#16213=ORIENTED_EDGE ( 'NONE', *, *, #4381, .T. ) ;
#16225=CARTESIAN_POINT ( 'NONE',  ( -8.699999999648399651, -15.36399602968765521, -37.98537634616555181 ) ) ;
#16245=EDGE_LOOP ( 'NONE', ( #22826, #14938, #9004, #3585 ) ) ;
#16255=CARTESIAN_POINT ( 'NONE',  ( -8.699999999628206027, -18.27232546675181268, -40.96725586010739306 ) ) ;
#16260=DIRECTION ( 'NONE',  ( -1.000000000000000000, 5.687697913155423197E-16, -6.771501495041734442E-12 ) ) ;
#16311=FACE_OUTER_BOUND ( 'NONE', #15943, .T. ) ;
#16334=EDGE_LOOP ( 'NONE', ( #2336, #14634, #1768, #8083 ) ) ;
#16338=CYLINDRICAL_SURFACE ( 'NONE', #24331, 2.500000000000000888 ) ;
#16352=CARTESIAN_POINT ( 'NONE',  ( -7.999999999628064629, -15.40335946066103645, -40.52613281826078406 ) ) ;
#16365=EDGE_CURVE ( 'NONE', #10911, #8911, #11093, .T. ) ;
#16369=EDGE_CURVE ( 'NONE', #13888, #29654, #27926, .T. ) ;
#16392=DIRECTION ( 'NONE',  ( 1.000000000000000000, -9.219999999999999084E-13, 4.710999999999999616E-12 ) ) ;
#16398=ORIENTED_EDGE ( 'NONE', *, *, #20888, .T. ) ;
#16411=( NAMED_UNIT ( * ) PLANE_ANGLE_UNIT ( ) SI_UNIT ( $, .RADIAN. ) );
#16425=CARTESIAN_POINT ( 'NONE',  ( -7.999999999695856623, -18.27877680370596636, -30.94409471158115110 ) ) ;
#16435=EDGE_CURVE ( 'NONE', #28713, #9163, #10101, .T. ) ;
#16438=CARTESIAN_POINT ( 'NONE',  ( 8.000000000250640397, -26.29778505802628885, -31.34318562232667915 ) ) ;
#16450=ORIENTED_EDGE ( 'NONE', *, *, #30180, .T. ) ;
#16466=CARTESIAN_POINT ( 'NONE',  ( 8.700000000231835173, -28.43890284012990577, -25.73830582827173785 ) ) ;
#16472=CARTESIAN_POINT ( 'NONE',  ( -8.000000000474178918, -29.73863906514523947, -27.17531388891475075 ) ) ;
#16509=CARTESIAN_POINT ( 'NONE',  ( 7.000000000277405654, -5.572998883592096497, -27.02754848641193419 ) ) ;
#16512=VECTOR ( 'NONE', #223, 1000.000000000000000 ) ;
#16555=ORIENTED_EDGE ( 'NONE', *, *, #30982, .T. ) ;
#16556=CARTESIAN_POINT ( 'NONE',  ( -5.797918471703387588, -5.490503403362547274, -26.84307236416243470 ) ) ;
#16591=DIRECTION ( 'NONE',  ( 1.000000000000000000, -1.843431230198065828E-12, 2.650498504953516580E-12 ) ) ;
#16602=CARTESIAN_POINT ( 'NONE',  ( -7.999999999693439889, -7.565603753653322272, -31.48340496202311911 ) ) ;
#16604=EDGE_CURVE ( 'NONE', #15836, #7991, #15001, .T. ) ;
#16606=VERTEX_POINT ( 'NONE', #19413 ) ;
#16613=CARTESIAN_POINT ( 'NONE',  ( 8.700000000115439391, -60.75400889061209142, -3.446705952623797309 ) ) ;
#16614=ORIENTED_EDGE ( 'NONE', *, *, #2412, .F. ) ;
#16629=ORIENTED_EDGE ( 'NONE', *, *, #13726, .T. ) ;
#16641=CARTESIAN_POINT ( 'NONE',  ( 8.699999999546083274, -16.84112679186181083, -33.19732076799427034 ) ) ;
#16653=B_SPLINE_CURVE_WITH_KNOTS ( 'NONE', 5,
 ( #11720, #23693, #2127, #26199, #21321, #14090, #4636, #16736, #7154 ),
 .UNSPECIFIED., .F., .F.,
 ( 6, 3, 6 ),
 ( 0.000000000000000000, 1.646696146390000060, 2.782752057450000205 ),
 .UNSPECIFIED. ) ;
#16657=DIRECTION ( 'NONE',  ( 1.000000000000000000, -1.843431230208684678E-12, 2.650498504958264790E-12 ) ) ;
#16666=CARTESIAN_POINT ( 'NONE',  ( -7.999999999651500993, -14.33807524410660328, -37.46575453387659849 ) ) ;
#16668=ORIENTED_EDGE ( 'NONE', *, *, #14444, .T. ) ;
#16675=ORIENTED_EDGE ( 'NONE', *, *, #17652, .T. ) ;
#16676=DIRECTION ( 'NONE',  ( -3.133604487004501508E-12, -0.3568421334038989756, 0.9341647027306019258 ) ) ;
#16692=LINE ( 'NONE', #4754, #22691 ) ;
#16702=DIRECTION ( 'NONE',  ( -0.7071067811842725037, -0.2886612846624971307, -0.6455034180701249014 ) ) ;
#16707=EDGE_LOOP ( 'NONE', ( #27392, #15462, #9554, #8189 ) ) ;
#16736=CARTESIAN_POINT ( 'NONE',  ( -7.999999999660801109, -18.34164001289334678, -36.27507178818978417 ) ) ;
#16761=LINE ( 'NONE', #7481, #17826 ) ;
#16779=CARTESIAN_POINT ( 'NONE',  ( -7.999999999729824118, -28.31424580201955621, -25.69835907506571715 ) ) ;
#16781=CARTESIAN_POINT ( 'NONE',  ( 7.707106507606773960, -115.2381290211091738, 21.69251943803729787 ) ) ;
#16786=DIRECTION ( 'NONE',  ( 0.000000000000000000, -0.9128796883888953273, 0.4082287037029526666 ) ) ;
#16792=VECTOR ( 'NONE', #10899, 1000.000000000000000 ) ;
#16817=EDGE_CURVE ( 'NONE', #4458, #8842, #19378, .T. ) ;
#16818=CARTESIAN_POINT ( 'NONE',  ( 8.000000000647496279, -17.71277672293419769, -33.66803003880371392 ) ) ;
#16823=CARTESIAN_POINT ( 'NONE',  ( 8.700000000245104559, -24.05709603917588524, -27.69722300140832871 ) ) ;
#16827=CARTESIAN_POINT ( 'NONE',  ( -7.999999999650268201, -15.05691661382650537, -37.86814300153927348 ) ) ;
#16828=MECHANICAL_DESIGN_GEOMETRIC_PRESENTATION_REPRESENTATION('',(#29380),#21358);
#16835=ORIENTED_EDGE ( 'NONE', *, *, #6074, .F. ) ;
#16844=DIRECTION ( 'NONE',  ( -1.000000000000000000, 5.687697913153403713E-16, -6.771501495041734442E-12 ) ) ;
#16865=LINE ( 'NONE', #21285, #25389 ) ;
#16882=VERTEX_POINT ( 'NONE', #22198 ) ;
#16886=CARTESIAN_POINT ( 'NONE',  ( -7.999999999650137639, -15.20668219507512653, -37.92535107952787854 ) ) ;
#16902=ORIENTED_EDGE ( 'NONE', *, *, #4405, .T. ) ;
#16913=B_SPLINE_CURVE_WITH_KNOTS ( 'NONE', 4,
 ( #14324, #9735, #16818, #9898, #23924 ),
 .UNSPECIFIED., .F., .F.,
 ( 5, 5 ),
 ( -0.9817477042479999527, 0.9817477042479999527 ),
 .UNSPECIFIED. ) ;
#16916=EDGE_CURVE ( 'NONE', #31008, #15988, #26459, .T. ) ;
#16921=VERTEX_POINT ( 'NONE', #12128 ) ;
#16927=CARTESIAN_POINT ( 'NONE',  ( -8.699999999723049271, -24.33803193940951104, -26.96176843113012112 ) ) ;
#16931=DIRECTION ( 'NONE',  ( 3.133604487004501912E-12, 0.3568421334038983650, -0.9341647027306021478 ) ) ;
#16986=ORIENTED_EDGE ( 'NONE', *, *, #30739, .T. ) ;
#16993=LINE ( 'NONE', #26288, #3494 ) ;
#17000=CARTESIAN_POINT ( 'NONE',  ( 8.700000000280658341, -13.90765988010977239, -34.05269868223890484 ) ) ;
#17003=CARTESIAN_POINT ( 'NONE',  ( -8.699999998930268319, -15.05691612485074948, -37.86814428179198444 ) ) ;
#17027=ORIENTED_EDGE ( 'NONE', *, *, #28054, .T. ) ;
#17033=VERTEX_POINT ( 'NONE', #8318 ) ;
#17044=ADVANCED_BREP_SHAPE_REPRESENTATION ( '', ( #438, #17722 ), #9278 ) ;
#17051=CARTESIAN_POINT ( 'NONE',  ( 8.000000000278095769, -14.92844969908619035, -33.25053330389217621 ) ) ;
#17052=CARTESIAN_POINT ( 'NONE',  ( 8.699999999555858565, -13.61360970152257721, -34.64062719131236179 ) ) ;
#17054=CARTESIAN_POINT ( 'NONE',  ( -7.999999999719110022, -29.98791861939423598, -27.92402217208466197 ) ) ;
#17069=VECTOR ( 'NONE', #18257, 1000.000000000000000 ) ;
#17072=CARTESIAN_POINT ( 'NONE',  ( 8.000000000252409649, -24.26136093482662304, -29.62468611105709471 ) ) ;
#17087=LINE ( 'NONE', #7641, #24319 ) ;
#17107=CARTESIAN_POINT ( 'NONE',  ( 8.000000000251251464, -25.56183060493181358, -31.06205794070631043 ) ) ;
#17111=CYLINDRICAL_SURFACE ( 'NONE', #10432, 3.000000000000002220 ) ;
#17114=EDGE_LOOP ( 'NONE', ( #11859, #9470, #16213, #1401 ) ) ;
#17124=CARTESIAN_POINT ( 'NONE',  ( -7.999999999945442752, -112.0649859495781300, 5.802913492026387843 ) ) ;
#17139=FACE_OUTER_BOUND ( 'NONE', #27877, .T. ) ;
#17154=DIRECTION ( 'NONE',  ( -1.000000000000000000, 5.687697999151106851E-16, -6.771501495036750356E-12 ) ) ;
#17167=ORIENTED_EDGE ( 'NONE', *, *, #21334, .T. ) ;
#17169=EDGE_CURVE ( 'NONE', #17596, #61, #7491, .T. ) ;
#17170=CARTESIAN_POINT ( 'NONE',  ( 8.000000000858760174, -25.41682687355206482, -25.82167197184731577 ) ) ;
#17176=FACE_OUTER_BOUND ( 'NONE', #27816, .T. ) ;
#17179=VERTEX_POINT ( 'NONE', #8797 ) ;
#17197=CYLINDRICAL_SURFACE ( 'NONE', #15480, 3.000000000000002220 ) ;
#17226=CARTESIAN_POINT ( 'NONE',  ( -7.999999999683915952, -16.84112630284391443, -33.19732204833458411 ) ) ;
#17241=AXIS2_PLACEMENT_3D ( 'NONE', #12745, #20145, #22975 ) ;
#17264=CARTESIAN_POINT ( 'NONE',  ( 8.700000000275174727, -18.43913150047637828, -35.13595876467604739 ) ) ;
#17277=CARTESIAN_POINT ( 'NONE',  ( -7.999999999984332533, -116.7459945346252113, 11.01907316483054622 ) ) ;
#17284=VECTOR ( 'NONE', #1787, 1000.000000000000000 ) ;
#17299=CARTESIAN_POINT ( 'NONE',  ( 8.000000000658319621, -14.18526619378945774, -37.39743501090877942 ) ) ;
#17301=CARTESIAN_POINT ( 'NONE',  ( -8.699999999715885224, -26.99999999997790923, -28.40000000002690683 ) ) ;
#17324=ORIENTED_EDGE ( 'NONE', *, *, #7436, .F. ) ;
#17332=CARTESIAN_POINT ( 'NONE',  ( -8.699999999692932917, -26.69041892758821888, -31.40984194557997000 ) ) ;
#17333=ORIENTED_EDGE ( 'NONE', *, *, #28604, .F. ) ;
#17342=DIRECTION ( 'NONE',  ( 1.000000000000000000, -1.843431230204166689E-12, 2.650498504954120002E-12 ) ) ;
#17362=CARTESIAN_POINT ( 'NONE',  ( -8.699999999662093586, -15.94902145834643115, -35.53273252493492862 ) ) ;
#17427=CARTESIAN_POINT ( 'NONE',  ( -8.699999999691694796, -25.92947359974585098, -31.20249410827203107 ) ) ;
#17436=EDGE_CURVE ( 'NONE', #15429, #1748, #27115, .T. ) ;
#17443=ORIENTED_EDGE ( 'NONE', *, *, #24537, .F. ) ;
#17453=DIRECTION ( 'NONE',  ( 1.000000000000000000, -1.843431230198065424E-12, 2.650498504953516580E-12 ) ) ;
#17480=CARTESIAN_POINT ( 'NONE',  ( 7.963158867438391297, -115.4064749715892617, 21.31606477568482916 ) ) ;
#17483=ORIENTED_EDGE ( 'NONE', *, *, #2753, .T. ) ;
#17488=ORIENTED_EDGE ( 'NONE', *, *, #14073, .F. ) ;
#17504=DIRECTION ( 'NONE',  ( -3.924189347185961537E-12, 0.4082287037029530552, 0.9128796883888952163 ) ) ;
#17525=VERTEX_POINT ( 'NONE', #12630 ) ;
#17538=DIRECTION ( 'NONE',  ( 1.666951178525963134E-12, -0.4082287037029531107, -0.9128796883888953273 ) ) ;
#17545=DIRECTION ( 'NONE',  ( -1.000000000000000000, 9.219999999999999084E-13, -4.710999999999999616E-12 ) ) ;
#17551=ORIENTED_EDGE ( 'NONE', *, *, #19531, .F. ) ;
#17575=LINE ( 'NONE', #19946, #11769 ) ;
#17589=AXIS2_PLACEMENT_3D ( 'NONE', #2532, #16844, #6936 ) ;
#17592=ORIENTED_EDGE ( 'NONE', *, *, #30970, .F. ) ;
#17593=LINE ( 'NONE', #20267, #15268 ) ;
#17596=VERTEX_POINT ( 'NONE', #8679 ) ;
#17600=CIRCLE ( 'NONE', #22136, 1.700000000000000178 ) ;
#17601=CARTESIAN_POINT ( 'NONE',  ( 8.000000000284819279, -13.66682223737133128, -36.55330428412179344 ) ) ;
#17616=DIRECTION ( 'NONE',  ( 2.966427579999808118E-12, 0.8902635789278698919, -0.4554456718803465143 ) ) ;
#17617=CARTESIAN_POINT ( 'NONE',  ( -8.699999999732469291, -28.77621036647359887, -25.95065533197870167 ) ) ;
#17625=VERTEX_POINT ( 'NONE', #23177 ) ;
#17635=CARTESIAN_POINT ( 'NONE',  ( -8.699999999693440955, -7.565603753652677455, -31.48340496202640892 ) ) ;
#17636=CARTESIAN_POINT ( 'NONE',  ( -7.999999999660042604, -18.28443193496838504, -36.42483736938474692 ) ) ;
#17641=CARTESIAN_POINT ( 'NONE',  ( -7.620434517381760919, -5.659705516265826297, -27.22144157413186250 ) ) ;
#17652=EDGE_CURVE ( 'NONE', #13180, #23040, #1617, .T. ) ;
#17656=ORIENTED_EDGE ( 'NONE', *, *, #28811, .F. ) ;
#17663=VERTEX_POINT ( 'NONE', #28039 ) ;
#17668=CARTESIAN_POINT ( 'NONE',  ( 7.999999999945623941, -115.1185614904247814, 21.95989595802063121 ) ) ;
#17701=CARTESIAN_POINT ( 'NONE',  ( -8.699999999703425857, -29.80249410822303346, -29.47052640025896508 ) ) ;
#17708=ORIENTED_EDGE ( 'NONE', *, *, #14486, .T. ) ;
#17712=CARTESIAN_POINT ( 'NONE',  ( 8.700000000287717583, -16.96959321760160222, -37.81493174583334849 ) ) ;
#17721=DIRECTION ( 'NONE',  ( 1.000000000000000000, -1.841917067661885521E-12, 2.653884470265303553E-12 ) ) ;
#17722=AXIS2_PLACEMENT_3D ( 'NONE', #2627, #14015, #29203 ) ;
#17748=CARTESIAN_POINT ( 'NONE',  ( 8.000000000289732682, -15.05691661385925961, -37.86814300156539304 ) ) ;
#17754=CARTESIAN_POINT ( 'NONE',  ( 8.699999999548097662, -14.92844969910509079, -33.25053330388070805 ) ) ;
#17766=CARTESIAN_POINT ( 'NONE',  ( -8.699999999733913469, -28.43737202012412624, -25.73763746937040864 ) ) ;
#17767=VECTOR ( 'NONE', #2399, 1000.000000000000000 ) ;
#17778=CARTESIAN_POINT ( 'NONE',  ( 7.989499821578848859, -115.4538843872006453, 21.21004799597932688 ) ) ;
#17794=VECTOR ( 'NONE', #15814, 999.9999999999998863 ) ;
#17805=CARTESIAN_POINT ( 'NONE',  ( 8.000000000252409649, -24.26136093482662304, -29.62468611105709471 ) ) ;
#17810=ORIENTED_EDGE ( 'NONE', *, *, #14607, .T. ) ;
#17826=VECTOR ( 'NONE', #14419, 1000.000000000000000 ) ;
#17844=CARTESIAN_POINT ( 'NONE',  ( 1.030019577584204020E-10, -102.7755780389355778, 17.20706796825876239 ) ) ;
#17863=CARTESIAN_POINT ( 'NONE',  ( 8.699999999531884853, -22.83323352251082738, -39.84673050073825351 ) ) ;
#17910=CARTESIAN_POINT ( 'NONE',  ( 8.000000000287716517, -16.96959321760095563, -37.81493174583665251 ) ) ;
#17914=FACE_OUTER_BOUND ( 'NONE', #16707, .T. ) ;
#17922=CARTESIAN_POINT ( 'NONE',  ( -7.999999999720831312, -24.33763747047824566, -26.96262797785872678 ) ) ;
#17944=CARTESIAN_POINT ( 'NONE',  ( -6.999999999262594308, -5.572998883415898774, -27.02754848611273530 ) ) ;
#17955=CARTESIAN_POINT ( 'NONE',  ( -8.000000000474178918, -29.73863906514523947, -27.17531388891475075 ) ) ;
#17979=CARTESIAN_POINT ( 'NONE',  ( -8.699999999630685821, -15.59624655979752461, -40.60108361767771612 ) ) ;
#17985=FACE_OUTER_BOUND ( 'NONE', #611, .T. ) ;
#17999=B_SPLINE_CURVE_WITH_KNOTS ( 'NONE', 4,
 ( #11098, #22903, #24791, #15648, #6051 ),
 .UNSPECIFIED., .F., .F.,
 ( 5, 5 ),
 ( -0.9817477042459999970, 0.9817477042459999970 ),
 .UNSPECIFIED. ) ;
#18002=VERTEX_POINT ( 'NONE', #8802 ) ;
#18003=CARTESIAN_POINT ( 'NONE',  ( 2.633098176678708328E-10, -9.034299563938168021, -24.71289265967806514 ) ) ;
#18004=CARTESIAN_POINT ( 'NONE',  ( -8.700000000030557956, -116.5561065468281186, 18.74526241736806043 ) ) ;
#18035=DIRECTION ( 'NONE',  ( -2.966427579999808118E-12, -0.8902635789278700029, 0.4554456718803465698 ) ) ;
#18036=DIRECTION ( 'NONE',  ( 1.000000000000000000, -1.843431230204166689E-12, 2.650498504954120002E-12 ) ) ;
#18057=B_SPLINE_CURVE_WITH_KNOTS ( 'NONE', 3,
 ( #17427, #12401, #28929, #9890, #14769, #14926 ),
 .UNSPECIFIED., .F., .F.,
 ( 4, 2, 4 ),
 ( 0.000000000000000000, 0.5000000000000000000, 1.000000000000000000 ),
 .UNSPECIFIED. ) ;
#18072=EDGE_CURVE ( 'NONE', #5252, #23079, #13429, .T. ) ;
#18079=CARTESIAN_POINT ( 'NONE',  ( 8.000000000355418805, -28.43737202112227536, -25.73763746985420653 ) ) ;
#18107=CARTESIAN_POINT ( 'NONE',  ( -7.999999999672612994, -13.51119859729762496, -34.94474744671868649 ) ) ;
#18109=ORIENTED_EDGE ( 'NONE', *, *, #6621, .T. ) ;
#18127=ORIENTED_EDGE ( 'NONE', *, *, #21960, .T. ) ;
#18128=ADVANCED_FACE ( 'NONE', ( #19027 ), #7069, .F. ) ;
#18135=EDGE_LOOP ( 'NONE', ( #8617, #29288, #10714, #16555, #15351 ) ) ;
#18145=CARTESIAN_POINT ( 'NONE',  ( -7.999999999691694619, -25.92947359974649046, -31.20249410826873415 ) ) ;
#18177=ORIENTED_EDGE ( 'NONE', *, *, #1443, .T. ) ;
#18186=EDGE_CURVE ( 'NONE', #21002, #24719, #13370, .T. ) ;
#18194=DIRECTION ( 'NONE',  ( -1.000000000000000000, 0.000000000000000000, -6.771289003360644742E-12 ) ) ;
#18197=CARTESIAN_POINT ( 'NONE',  ( -6.999999999884560786, -60.75400889059761766, -3.446705952697758590 ) ) ;
#18200=DIRECTION ( 'NONE',  ( 8.579942312181285869E-13, 0.9431856258987900699, 0.3322662713817151059 ) ) ;
#18220=PLANE ( 'NONE',  #15447 ) ;
#18221=CARTESIAN_POINT ( 'NONE',  ( -7.999999999718669486, -5.981227587262960554, -27.94042817487965991 ) ) ;
#18224=LINE ( 'NONE', #13193, #21029 ) ;
#18250=DIRECTION ( 'NONE',  ( 3.924189347185962345E-12, -0.4082287037029530552, -0.9128796883888953273 ) ) ;
#18257=DIRECTION ( 'NONE',  ( -1.000000000000000000, 5.687697999151106851E-16, -6.771501495036750356E-12 ) ) ;
#18270=VECTOR ( 'NONE', #30768, 1000.000000000000000 ) ;
#18297=ORIENTED_EDGE ( 'NONE', *, *, #4894, .F. ) ;
#18302=( NAMED_UNIT ( * ) PLANE_ANGLE_UNIT ( ) SI_UNIT ( $, .RADIAN. ) );
#18307=CARTESIAN_POINT ( 'NONE',  ( -8.699999999628362346, -14.95623164695839513, -40.37561726986208299 ) ) ;
#18310=CARTESIAN_POINT ( 'NONE',  ( -7.999999999692273711, -26.69088343935172958, -31.40976070826679489 ) ) ;
#18322=CARTESIAN_POINT ( 'NONE',  ( -8.699999998983425797, -29.80249410822303346, -29.47052640025896508 ) ) ;
#18325=AXIS2_PLACEMENT_3D ( 'NONE', #14216, #2868, #28990 ) ;
#18331=DIRECTION ( 'NONE',  ( 1.000000000000000000, -1.843431230198065424E-12, 2.650498504953516580E-12 ) ) ;
#18333=LINE ( 'NONE', #18641, #24347 ) ;
#18341=CARTESIAN_POINT ( 'NONE',  ( 7.801126876359127493, -5.730966291675875013, -27.38079468629169355 ) ) ;
#18357=CARTESIAN_POINT ( 'NONE',  ( -8.699999999660043670, -18.28443321518998133, -36.42483785847389299 ) ) ;
#18368=CARTESIAN_POINT ( 'NONE',  ( -8.699999998935181722, -13.66682223737418944, -36.55330428419230060 ) ) ;
#18369=DIRECTION ( 'NONE',  ( 1.667044707805962905E-12, -0.4082287037029530552, -0.9128796883888953273 ) ) ;
#18386=VERTEX_POINT ( 'NONE', #24625 ) ;
#18395=CARTESIAN_POINT ( 'NONE',  ( 8.000000000279957391, -18.28443193505134445, -36.42483736938841332 ) ) ;
#18423=LINE ( 'NONE', #13389, #24115 ) ;
#18438=CARTESIAN_POINT ( 'NONE',  ( -7.999999999722595234, -5.572998883578264895, -27.02754848648259767 ) ) ;
#18444=EDGE_LOOP ( 'NONE', ( #30022, #9324, #10335, #1900 ) ) ;
#18462=EDGE_CURVE ( 'NONE', #4458, #15161, #21638, .T. ) ;
#18484=ADVANCED_FACE ( 'NONE', ( #12823 ), #24163, .F. ) ;
#18489=CARTESIAN_POINT ( 'NONE',  ( -8.700000000022731328, -117.0726643331094152, 17.59013758954728246 ) ) ;
#18492=VECTOR ( 'NONE', #21939, 1000.000000000000000 ) ;
#18501=ORIENTED_EDGE ( 'NONE', *, *, #11718, .F. ) ;
#18505=EDGE_LOOP ( 'NONE', ( #9207, #23499, #18127, #10175 ) ) ;
#18518=DIRECTION ( 'NONE',  ( -1.000000000000000000, 5.687697999151106851E-16, -6.771501495036750356E-12 ) ) ;
#18529=CARTESIAN_POINT ( 'NONE',  ( -8.699999999715885224, -26.99999999997790923, -28.40000000002690683 ) ) ;
#18578=ORIENTED_EDGE ( 'NONE', *, *, #9471, .F. ) ;
#18613=EDGE_LOOP ( 'NONE', ( #14870, #20069, #24801, #17551, #3600, #29059, #17443, #14945 ) ) ;
#18622=CARTESIAN_POINT ( 'NONE',  ( 8.000000000860607585, -29.89895010222698701, -27.53380090417111958 ) ) ;
#18632=CARTESIAN_POINT ( 'NONE',  ( -7.999999999975165643, -111.9817663810327275, 5.760339591561383088 ) ) ;
#18641=CARTESIAN_POINT ( 'NONE',  ( 4.276011752470107119, -42.94729992904354532, -9.547410993441516780 ) ) ;
#18651=CARTESIAN_POINT ( 'NONE',  ( -7.999999999730073696, -28.07052495761531219, -25.59750966829892960 ) ) ;
#18736=CARTESIAN_POINT ( 'NONE',  ( 8.700000000278567569, -14.35781456214690266, -33.57689241567665306 ) ) ;
#18749=CIRCLE ( 'NONE', #2182, 4.276011752367109509 ) ;
#18758=DIRECTION ( 'NONE',  ( -3.924189347185962345E-12, 0.4082287037029531107, 0.9128796883888953273 ) ) ;
#18768=CARTESIAN_POINT ( 'NONE',  ( -8.699999999642283655, -16.96959321760381556, -37.81493174590716677 ) ) ;
#18774=DIRECTION ( 'NONE',  ( 2.764840495839172514E-12, 0.9128796883888952163, -0.4082287037029530552 ) ) ;
#18789=DIRECTION ( 'NONE',  ( 0.000000000000000000, -0.9128796883888953273, 0.4082287037029528332 ) ) ;
#18790=CARTESIAN_POINT ( 'NONE',  ( 8.000000000247633025, -27.86541989009443654, -31.29929855349184464 ) ) ;
#18791=VECTOR ( 'NONE', #29509, 999.9999999999998863 ) ;
#18802=ORIENTED_EDGE ( 'NONE', *, *, #17436, .F. ) ;
#18806=ORIENTED_EDGE ( 'NONE', *, *, #28306, .T. ) ;
#18818=DIRECTION ( 'NONE',  ( -6.326189572192214457E-12, -0.3568421334038989756, 0.9341647027306019258 ) ) ;
#18821=EDGE_CURVE ( 'NONE', #10703, #12816, #22470, .T. ) ;
#18826=B_SPLINE_CURVE_WITH_KNOTS ( 'NONE', 3,
 ( #21846, #17107, #19166, #21998, #28611, #19326 ),
 .UNSPECIFIED., .F., .F.,
 ( 4, 2, 4 ),
 ( 0.000000000000000000, 0.5000000000000000000, 1.000000000000000000 ),
 .UNSPECIFIED. ) ;
#18833=CARTESIAN_POINT ( 'NONE',  ( 4.276011752472853367, -43.23306002163561601, -10.18642677531374829 ) ) ;
#18864=EDGE_CURVE ( 'NONE', #27730, #1828, #30268, .T. ) ;
#18870=CARTESIAN_POINT ( 'NONE',  ( -7.999999999635500458, -22.00621177641532000, -40.24039824850300562 ) ) ;
#18877=PRODUCT_DEFINITION_FORMATION_WITH_SPECIFIED_SOURCE ( 'ANY', '', #13934, .NOT_KNOWN. ) ;
#18893=EDGE_LOOP ( 'NONE', ( #14936, #23625, #10877, #27198 ) ) ;
#18915=ADVANCED_FACE ( 'NONE', ( #20567 ), #23418, .T. ) ;
#18937=VECTOR ( 'NONE', #256, 999.9999999999998863 ) ;
#18939=CARTESIAN_POINT ( 'NONE',  ( -7.999999999650066584, -15.36103638014619222, -37.97055538590272761 ) ) ;
#18941=ORIENTED_EDGE ( 'NONE', *, *, #27247, .F. ) ;
#18946=CARTESIAN_POINT ( 'NONE',  ( 7.999999999489548763, -115.5267901939644446, 21.04701626999689168 ) ) ;
#18953=LINE ( 'NONE', #23846, #13089 ) ;
#18978=EDGE_CURVE ( 'NONE', #23086, #22033, #6558, .T. ) ;
#19001=VERTEX_POINT ( 'NONE', #6085 ) ;
#19009=ADVANCED_FACE ( 'NONE', ( #4202 ), #30647, .F. ) ;
#19027=FACE_OUTER_BOUND ( 'NONE', #26876, .T. ) ;
#19075=CYLINDRICAL_SURFACE ( 'NONE', #10269, 4.276011752367109509 ) ;
#19079=EDGE_CURVE ( 'NONE', #19543, #18386, #15594, .T. ) ;
#19083=ORIENTED_EDGE ( 'NONE', *, *, #23329, .F. ) ;
#19096=ORIENTED_EDGE ( 'NONE', *, *, #5628, .F. ) ;
#19150=FACE_OUTER_BOUND ( 'NONE', #25549, .T. ) ;
#19159=VERTEX_POINT ( 'NONE', #14586 ) ;
#19166=CARTESIAN_POINT ( 'NONE',  ( 8.000000000251308307, -25.22417743378453281, -30.84961367804113763 ) ) ;
#19183=CARTESIAN_POINT ( 'NONE',  ( -7.999999999946012075, -112.2299448184148645, 5.890987397396584946 ) ) ;
#19202=ORIENTED_EDGE ( 'NONE', *, *, #18978, .F. ) ;
#19228=CARTESIAN_POINT ( 'NONE',  ( -7.999999999668361284, -14.95611408987656965, -40.37595097054163773 ) ) ;
#19254=CARTESIAN_POINT ( 'NONE',  ( -7.999999999651103977, -16.53431405373043717, -37.98000797241422788 ) ) ;
#19276=ORIENTED_EDGE ( 'NONE', *, *, #21630, .F. ) ;
#19303=DIRECTION ( 'NONE',  ( 1.000000000000000000, -1.843431230208684678E-12, 2.650498504958264790E-12 ) ) ;
#19319=ORIENTED_EDGE ( 'NONE', *, *, #8289, .T. ) ;
#19323=EDGE_LOOP ( 'NONE', ( #29340, #12920, #2445, #25906, #14287, #20627, #4677, #29561 ) ) ;
#19326=CARTESIAN_POINT ( 'NONE',  ( 8.000000000252409649, -24.26136093482662304, -29.62468611105709471 ) ) ;
#19338=LINE ( 'NONE', #19493, #31095 ) ;
#19349=ORIENTED_EDGE ( 'NONE', *, *, #21334, .F. ) ;
#19353=CARTESIAN_POINT ( 'NONE',  ( -7.999999999650885485, -14.58667674272277104, -37.64499445460491245 ) ) ;
#19358=ORIENTED_EDGE ( 'NONE', *, *, #15634, .F. ) ;
#19360=ORIENTED_EDGE ( 'NONE', *, *, #12124, .F. ) ;
#19361=CARTESIAN_POINT ( 'NONE',  ( -7.999999999730243339, -27.87661103596576595, -25.52343706782910360 ) ) ;
#19363=AXIS2_PLACEMENT_3D ( 'NONE', #16556, #14674, #2404 ) ;
#19366=CYLINDRICAL_SURFACE ( 'NONE', #2924, 3.000000000000002220 ) ;
#19376=CARTESIAN_POINT ( 'NONE',  ( 7.707106781468556100, -5.692566302608600637, -27.29492475672613594 ) ) ;
#19378=LINE ( 'NONE', #24410, #23238 ) ;
#19388=CARTESIAN_POINT ( 'NONE',  ( 8.000000000365092845, -24.33763746989997401, -26.96262797881743367 ) ) ;
#19394=ORIENTED_EDGE ( 'NONE', *, *, #29212, .T. ) ;
#19400=CARTESIAN_POINT ( 'NONE',  ( -8.699999999650268379, -15.05691612485074948, -37.86814428179198444 ) ) ;
#19401=CARTESIAN_POINT ( 'NONE',  ( -7.999999999669004325, -18.23122067930106027, -34.51216076568240965 ) ) ;
#19413=CARTESIAN_POINT ( 'NONE',  ( 8.000000000241653808, -24.19750966826863348, -27.32947504231146851 ) ) ;
#19421=ORIENTED_EDGE ( 'NONE', *, *, #17436, .T. ) ;
#19427=EDGE_CURVE ( 'NONE', #22839, #2756, #10696, .T. ) ;
#19431=CARTESIAN_POINT ( 'NONE',  ( 8.000000000236575204, -29.80249033211431708, -29.47052495773638370 ) ) ;
#19444=EDGE_CURVE ( 'NONE', #27730, #30584, #3606, .T. ) ;
#19458=EDGE_CURVE ( 'NONE', #6463, #16100, #22357, .T. ) ;
#19462=DIRECTION ( 'NONE',  ( 1.000000000000000000, -1.843431230208684274E-12, 2.650498504958264790E-12 ) ) ;
#19474=CARTESIAN_POINT ( 'NONE',  ( 8.700000000232448016, -27.70277699884391964, -25.45709603910293595 ) ) ;
#19476=ORIENTED_EDGE ( 'NONE', *, *, #25238, .F. ) ;
#19486=DIRECTION ( 'NONE',  ( 0.000000000000000000, -0.9128796883888949942, 0.4082287037029534438 ) ) ;
#19489=CYLINDRICAL_SURFACE ( 'NONE', #7261, 2.500000000000000888 ) ;
#19493=CARTESIAN_POINT ( 'NONE',  ( -7.707106781077335711, -60.46534760592810898, -2.801202534621561657 ) ) ;
#19508=CARTESIAN_POINT ( 'NONE',  ( -7.999999999652088967, -14.16511107073194076, -37.30738323264701251 ) ) ;
#19512=VERTEX_POINT ( 'NONE', #23455 ) ;
#19531=EDGE_CURVE ( 'NONE', #15161, #10063, #11097, .T. ) ;
#19543=VERTEX_POINT ( 'NONE', #2357 ) ;
#19549=CARTESIAN_POINT ( 'NONE',  ( 7.999999999489548763, -115.5267901939644446, 21.04701626999689168 ) ) ;
#19574=CARTESIAN_POINT ( 'NONE',  ( -4.276011752264103016, -42.94729992905724458, -9.547410993472153606 ) ) ;
#19580=CYLINDRICAL_SURFACE ( 'NONE', #24372, 2.500000000000000888 ) ;
#19594=LINE ( 'NONE', #99, #18937 ) ;
#19599=CARTESIAN_POINT ( 'NONE',  ( -7.999999999628841785, -14.30188212870945286, -40.14546951504663497 ) ) ;
#19600=CARTESIAN_POINT ( 'NONE',  ( -7.999999999683302221, -15.48251719072922050, -33.06200388856654371 ) ) ;
#19637=CARTESIAN_POINT ( 'NONE',  ( 1.057488903014505443E-10, -43.23306002164246564, -10.18642677532906049 ) ) ;
#19657=ORIENTED_EDGE ( 'NONE', *, *, #16171, .T. ) ;
#19668=CARTESIAN_POINT ( 'NONE',  ( -7.999999999727707589, -25.79195116312516589, -25.65395878494778259 ) ) ;
#19672=EDGE_CURVE ( 'NONE', #25555, #90, #4301, .T. ) ;
#19684=CARTESIAN_POINT ( 'NONE',  ( -8.699999998951904345, -14.92844969908904851, -33.25053330396269047 ) ) ;
#19693=ORIENTED_EDGE ( 'NONE', *, *, #11718, .T. ) ;
#19714=CARTESIAN_POINT ( 'NONE',  ( -7.707106507371444870, -5.692566414263196428, -27.29492500646317765 ) ) ;
#19725=CARTESIAN_POINT ( 'NONE',  ( -8.699999999724179034, -29.73863906514459643, -27.17531388891805477 ) ) ;
#19753=CARTESIAN_POINT ( 'NONE',  ( -7.999999999668208517, -9.149979920084513552, -35.02638174925785819 ) ) ;
#19761=DIRECTION ( 'NONE',  ( 1.000000000000000000, 1.601966730286663379E-12, 3.582312748438143944E-12 ) ) ;
#19771=CARTESIAN_POINT ( 'NONE',  ( -7.999999999681125296, -14.69158818474954487, -33.36927661519188604 ) ) ;
#19811=AXIS2_PLACEMENT_3D ( 'NONE', #22440, #5894, #12984 ) ;
#19822=ORIENTED_EDGE ( 'NONE', *, *, #1016, .T. ) ;
#19823=ORIENTED_EDGE ( 'NONE', *, *, #27247, .T. ) ;
#19827=ORIENTED_EDGE ( 'NONE', *, *, #18864, .T. ) ;
#19833=ADVANCED_FACE ( 'NONE', ( #8439 ), #8922, .T. ) ;
#19848=CARTESIAN_POINT ( 'NONE',  ( -8.000000000050450311, -115.5267901941129907, 21.04701626955636939 ) ) ;
#19862=CARTESIAN_POINT ( 'NONE',  ( -8.699999999693382335, -26.29778505801089850, -31.34318562240535044 ) ) ;
#19868=ORIENTED_EDGE ( 'NONE', *, *, #13147, .T. ) ;
#19875=DIRECTION ( 'NONE',  ( -3.582312748438143944E-12, 0.000000000000000000, 1.000000000000000000 ) ) ;
#19881=CARTESIAN_POINT ( 'NONE',  ( -8.699999999703425857, -29.80249410822303346, -29.47052640025896508 ) ) ;
#19890=CARTESIAN_POINT ( 'NONE',  ( -7.999999999711121745, -29.94262568603332042, -29.10368078042601780 ) ) ;
#19898=B_SPLINE_CURVE_WITH_KNOTS ( 'NONE', 3,
 ( #26106, #26257, #4695, #17264, #26871, #10503 ),
 .UNSPECIFIED., .F., .F.,
 ( 4, 2, 4 ),
 ( 0.000000000000000000, 0.5000000000000000000, 1.000000000000000000 ),
 .UNSPECIFIED. ) ;
#19899=ORIENTED_EDGE ( 'NONE', *, *, #20258, .T. ) ;
#19901=CARTESIAN_POINT ( 'NONE',  ( -8.000000000022961189, -117.2164086036294890, 17.00415548048141545 ) ) ;
#19902=EDGE_LOOP ( 'NONE', ( #26701, #5680, #6512, #5482 ) ) ;
#19908=ORIENTED_EDGE ( 'NONE', *, *, #28548, .T. ) ;
#19911=DIRECTION ( 'NONE',  ( 1.000000000000000000, -9.219999999999999084E-13, 4.710999999999999616E-12 ) ) ;
#19919=CARTESIAN_POINT ( 'NONE',  ( -8.699999999737658030, -25.77531388886905006, -25.66136093486021608 ) ) ;
#19934=CARTESIAN_POINT ( 'NONE',  ( 8.700000000290945223, -18.27255887617201324, -40.96732049143839305 ) ) ;
#19946=CARTESIAN_POINT ( 'NONE',  ( 8.350000000049549342, -115.5267901939647857, 21.04701626999854369 ) ) ;
#19953=CARTESIAN_POINT ( 'NONE',  ( 8.700000000272730460, -17.14815999457695028, -33.31467482405556524 ) ) ;
#19964=CARTESIAN_POINT ( 'NONE',  ( -8.699999999681903518, -14.92844969908904851, -33.25053330396269047 ) ) ;
#19970=VERTEX_POINT ( 'NONE', #18833 ) ;
#19971=EDGE_LOOP ( 'NONE', ( #26904, #19358, #4567, #12152, #1280, #7128, #29017, #13498 ) ) ;
#19975=CARTESIAN_POINT ( 'NONE',  ( 8.699999999525887873, -28.22468611110281245, -31.13863906511161517 ) ) ;
#19994=CARTESIAN_POINT ( 'NONE',  ( -7.999999999945165641, -111.9817663798748981, 5.760339591700875950 ) ) ;
#20011=CARTESIAN_POINT ( 'NONE',  ( 8.700000000248609311, -25.56262797786018837, -31.06236252946161969 ) ) ;
#20012=CARTESIAN_POINT ( 'NONE',  ( -7.999999999683915952, -16.84112630284391443, -33.19732204833458411 ) ) ;
#20067=LINE ( 'NONE', #3528, #2957 ) ;
#20069=ORIENTED_EDGE ( 'NONE', *, *, #18186, .T. ) ;
#20113=CARTESIAN_POINT ( 'NONE',  ( 8.700000000272682499, -17.42905530085155519, -33.49137094649729107 ) ) ;
#20120=EDGE_CURVE ( 'NONE', #7730, #27863, #29801, .T. ) ;
#20124=ORIENTED_EDGE ( 'NONE', *, *, #1016, .F. ) ;
#20125=DIRECTION ( 'NONE',  ( -6.181427515845962162E-12, 0.4082287037029531107, 0.9128796883888953273 ) ) ;
#20131=ORIENTED_EDGE ( 'NONE', *, *, #29489, .T. ) ;
#20135=CARTESIAN_POINT ( 'NONE',  ( 8.000000000287716517, -16.96959321760095563, -37.81493174583665251 ) ) ;
#20145=DIRECTION ( 'NONE',  ( 1.000000000000000000, -1.843431230200657634E-12, 2.650498504950726461E-12 ) ) ;
#20158=CARTESIAN_POINT ( 'NONE',  ( -8.000000000457589522, -24.26136093481186862, -29.62468611113247263 ) ) ;
#20203=EDGE_CURVE ( 'NONE', #12111, #23341, #8405, .T. ) ;
#20207=CARTESIAN_POINT ( 'NONE',  ( -8.699999999888484936, -60.34578018689309431, -2.533826264316873189 ) ) ;
#20209=EDGE_CURVE ( 'NONE', #30177, #3946, #20785, .T. ) ;
#20218=DIRECTION ( 'NONE',  ( -1.000000000000000000, 1.843431230205392516E-12, -2.650498504954667282E-12 ) ) ;
#20238=DIRECTION ( 'NONE',  ( -6.181333986565961785E-12, 0.4082287037029530552, 0.9128796883888953273 ) ) ;
#20258=EDGE_CURVE ( 'NONE', #22923, #28198, #16653, .T. ) ;
#20267=CARTESIAN_POINT ( 'NONE',  ( -8.000000000035504044, -116.0414483704504676, 19.89613934350951041 ) ) ;
#20274=ORIENTED_EDGE ( 'NONE', *, *, #14092, .T. ) ;
#20278=DIRECTION ( 'NONE',  ( 1.000000000000000000, -1.843431230200084908E-12, 2.650498504963248473E-12 ) ) ;
#20287=AXIS2_PLACEMENT_3D ( 'NONE', #28554, #4333, #2124 ) ;
#20291=CARTESIAN_POINT ( 'NONE',  ( -8.000000000050963678, -115.4736671374892722, 21.16580987455534668 ) ) ;
#20299=EDGE_CURVE ( 'NONE', #9121, #24850, #18953, .T. ) ;
#20301=EDGE_LOOP ( 'NONE', ( #27398, #11702, #24582, #4514 ) ) ;
#20306=CARTESIAN_POINT ( 'NONE',  ( 8.000000000289732682, -15.05691661385925961, -37.86814300156539304 ) ) ;
#20311=ORIENTED_EDGE ( 'NONE', *, *, #30210, .T. ) ;
#20330=B_SPLINE_CURVE_WITH_KNOTS ( 'NONE', 3,
 ( #13684, #14001, #25656, #6441, #30202, #21085 ),
 .UNSPECIFIED., .F., .F.,
 ( 4, 2, 4 ),
 ( 0.000000000000000000, 0.5000000000000000000, 1.000000000000000000 ),
 .UNSPECIFIED. ) ;
#20352=CARTESIAN_POINT ( 'NONE',  ( -6.999999999265341444, -5.287238791109590608, -26.38853270487952685 ) ) ;
#20355=FACE_OUTER_BOUND ( 'NONE', #22382, .T. ) ;
#20398=CARTESIAN_POINT ( 'NONE',  ( 8.700000000281498558, -22.22877482711028563, -40.15596262314623033 ) ) ;
#20399=EDGE_CURVE ( 'NONE', #26338, #27598, #896, .T. ) ;
#20424=ORIENTED_EDGE ( 'NONE', *, *, #1113, .F. ) ;
#20429=ORIENTED_EDGE ( 'NONE', *, *, #12551, .T. ) ;
#20448=CARTESIAN_POINT ( 'NONE',  ( 8.700000000277906764, -15.94902145836247342, -35.53273252485295330 ) ) ;
#20453=CARTESIAN_POINT ( 'NONE',  ( 8.000000000481156448, -28.77621036719994763, -25.95065533245048428 ) ) ;
#20457=CARTESIAN_POINT ( 'NONE',  ( -7.999999999726984612, -25.09035620932252186, -26.05319937760163285 ) ) ;
#20459=ORIENTED_EDGE ( 'NONE', *, *, #18186, .F. ) ;
#20480=CARTESIAN_POINT ( 'NONE',  ( -7.999999999669955564, -13.42967257572369277, -35.49331476339211378 ) ) ;
#20517=CARTESIAN_POINT ( 'NONE',  ( -7.999999999692422925, -27.47597782790758814, -31.38791861944036654 ) ) ;
#20519=CARTESIAN_POINT ( 'NONE',  ( 8.699999999974995291, -116.4387282421506029, 10.14683980968718835 ) ) ;
#20538=FACE_BOUND ( 'NONE', #13031, .T. ) ;
#20567=FACE_OUTER_BOUND ( 'NONE', #14679, .T. ) ;
#20589=LINE ( 'NONE', #15876, #28831 ) ;
#20591=CARTESIAN_POINT ( 'NONE',  ( -7.999999999703424791, -29.80249410822368006, -29.47052640025566816 ) ) ;
#20605=CARTESIAN_POINT ( 'NONE',  ( 8.000000000301639602, -14.95611408989132052, -40.37595097046627046 ) ) ;
#20614=CARTESIAN_POINT ( 'NONE',  ( -8.000000000477658801, -25.77531388886969310, -25.66136093485691916 ) ) ;
#20627=ORIENTED_EDGE ( 'NONE', *, *, #30294, .F. ) ;
#20654=EDGE_CURVE ( 'NONE', #11991, #13180, #6480, .T. ) ;
#20658=B_SPLINE_CURVE_WITH_KNOTS ( 'NONE', 3,
 ( #812, #25026, #6296, #30050, #27529, #3152 ),
 .UNSPECIFIED., .F., .F.,
 ( 4, 2, 4 ),
 ( 0.000000000000000000, 0.5000000000000000000, 1.000000000000000000 ),
 .UNSPECIFIED. ) ;
#20660=ORIENTED_EDGE ( 'NONE', *, *, #13898, .T. ) ;
#20664=ADVANCED_FACE ( 'NONE', ( #6330 ), #4287, .T. ) ;
#20665=CARTESIAN_POINT ( 'NONE',  ( 7.999999999994834354, -111.9817663810474642, 5.760339591636753021 ) ) ;
#20671=ORIENTED_EDGE ( 'NONE', *, *, #10344, .T. ) ;
#20685=FACE_OUTER_BOUND ( 'NONE', #17114, .T. ) ;
#20703=CARTESIAN_POINT ( 'NONE',  ( 8.699999999522411542, -24.26136093482726608, -29.62468611105379779 ) ) ;
#20726=ADVANCED_FACE ( 'NONE', ( #11833 ), #11673, .T. ) ;
#20731=CARTESIAN_POINT ( 'NONE',  ( 8.700000000111513643, -60.34578018690913837, -2.533826264234904091 ) ) ;
#20739=CYLINDRICAL_SURFACE ( 'NONE', #26813, 3.000000000000002220 ) ;
#20748=SURFACE_STYLE_USAGE ( .BOTH. , #6276 ) ;
#20762=CARTESIAN_POINT ( 'NONE',  ( 8.000000000232340369, -25.77531388888444752, -25.66136093478154123 ) ) ;
#20785=B_SPLINE_CURVE_WITH_KNOTS ( 'NONE', 3,
 ( #18004, #18489, #28087, #6533, #16129, #25741 ),
 .UNSPECIFIED., .F., .F.,
 ( 4, 2, 4 ),
 ( 0.000000000000000000, 0.5000000000000000000, 1.000000000000000000 ),
 .UNSPECIFIED. ) ;
#20796=VECTOR ( 'NONE', #27963, 1000.000000000000000 ) ;
#20808=EDGE_CURVE ( 'NONE', #21002, #3946, #16692, .T. ) ;
#20810=CARTESIAN_POINT ( 'NONE',  ( 6.999999999944251705, -114.9756814442911264, 22.27940384858688816 ) ) ;
#20832=EDGE_LOOP ( 'NONE', ( #26594, #3022, #19394, #19823, #8555, #29329, #28323, #25236 ) ) ;
#20839=CARTESIAN_POINT ( 'NONE',  ( 8.000000000236575204, -29.80249033211431708, -29.47052495773638370 ) ) ;
#20848=B_SPLINE_CURVE_WITH_KNOTS ( 'NONE', 3,
 ( #24256, #17922, #15275, #20457, #3461, #20614 ),
 .UNSPECIFIED., .F., .F.,
 ( 4, 2, 4 ),
 ( 0.000000000000000000, 0.5000000000000000000, 1.000000000000000000 ),
 .UNSPECIFIED. ) ;
#20849=AXIS2_PLACEMENT_3D ( 'NONE', #26122, #11641, #30838 ) ;
#20852=CARTESIAN_POINT ( 'NONE',  ( -8.699999998974114135, -28.22468611108677194, -31.13863906519358693 ) ) ;
#20855=CARTESIAN_POINT ( 'NONE',  ( -8.699999999684472130, -15.22718887828181522, -33.11694077318242790 ) ) ;
#20861=CARTESIAN_POINT ( 'NONE',  ( 8.000000000245886866, -28.22468611110216230, -31.13863906511491209 ) ) ;
#20888=EDGE_CURVE ( 'NONE', #22622, #27055, #24712, .T. ) ;
#20895=CARTESIAN_POINT ( 'NONE',  ( 8.700000000134913591, -66.94093258036980387, -17.28188441695247235 ) ) ;
#20908=ORIENTED_EDGE ( 'NONE', *, *, #29648, .F. ) ;
#20914=DIRECTION ( 'NONE',  ( 7.764622278472185525E-13, 0.9341647027306024809, 0.3568421334038978099 ) ) ;
#20915=PLANE ( 'NONE',  #6437 ) ;
#20943=ORIENTED_EDGE ( 'NONE', *, *, #20981, .F. ) ;
#20946=LINE ( 'NONE', #1446, #17069 ) ;
#20952=CARTESIAN_POINT ( 'NONE',  ( -8.699999999648149185, -16.34590724145236251, -38.02265883393443602 ) ) ;
#20972=VERTEX_POINT ( 'NONE', #20605 ) ;
#20973=LINE ( 'NONE', #19228, #17767 ) ;
#20981=EDGE_CURVE ( 'NONE', #27055, #23754, #14143, .T. ) ;
#20992=FACE_OUTER_BOUND ( 'NONE', #19902, .T. ) ;
#21002=VERTEX_POINT ( 'NONE', #21086 ) ;
#21029=VECTOR ( 'NONE', #954, 1000.000000000000000 ) ;
#21032=EDGE_LOOP ( 'NONE', ( #20131, #29717, #19822, #3621, #857 ) ) ;
#21042=EDGE_LOOP ( 'NONE', ( #2259, #22492, #19083, #30269 ) ) ;
#21075=CARTESIAN_POINT ( 'NONE',  ( -4.276011752261355880, -103.0613381315345123, 16.56805218637121513 ) ) ;
#21085=CARTESIAN_POINT ( 'NONE',  ( -8.000000000444114079, -28.22468611108740788, -31.13863906519029001 ) ) ;
#21086=CARTESIAN_POINT ( 'NONE',  ( -7.999999999985950794, -116.8591659214701792, 11.34031266722930908 ) ) ;
#21135=CYLINDRICAL_SURFACE ( 'NONE', #22378, 1.000000000000001332 ) ;
#21155=ORIENTED_EDGE ( 'NONE', *, *, #29397, .T. ) ;
#21178=CARTESIAN_POINT ( 'NONE',  ( -7.999999999638116144, -22.83323352248630655, -39.84673050082100332 ) ) ;
#21181=CARTESIAN_POINT ( 'NONE',  ( 8.000000000229924524, -28.07052495763006661, -25.59750966822355522 ) ) ;
#21215=CARTESIAN_POINT ( 'NONE',  ( -8.699999999952064300, -113.1082736028020577, 6.336644014756059207 ) ) ;
#21282=CARTESIAN_POINT ( 'NONE',  ( 8.700000000275743162, -15.22877080015275908, -33.11623335687269076 ) ) ;
#21285=CARTESIAN_POINT ( 'NONE',  ( 8.699999999516576210, -29.80249410823907752, -29.47052640017699687 ) ) ;
#21286=LINE ( 'NONE', #9319, #28856 ) ;
#21287=ORIENTED_EDGE ( 'NONE', *, *, #14968, .T. ) ;
#21290=SHAPE_REPRESENTATION_RELATIONSHIP ( 'NONE' , 'NONE' ,  #24039, #17044 ) ;
#21293=B_SPLINE_CURVE_WITH_KNOTS ( 'NONE', 3,
 ( #9845, #21967, #14263, #26828, #4966, #23869, #14578, #2310, #419, #24165 ),
 .UNSPECIFIED., .F., .F.,
 ( 4, 2, 2, 2, 4 ),
 ( 0.000000000000000000, 0.2500000000000000000, 0.5000000000000000000, 0.7500000000000000000, 1.000000000000000000 ),
 .UNSPECIFIED. ) ;
#21321=CARTESIAN_POINT ( 'NONE',  ( -7.999999999664230366, -18.46837034096498442, -35.57215028647357968 ) ) ;
#21330=VERTEX_POINT ( 'NONE', #15857 ) ;
#21334=EDGE_CURVE ( 'NONE', #8037, #16, #12796, .T. ) ;
#21342=CARTESIAN_POINT ( 'NONE',  ( 7.999999999977091214, -107.4273096626279482, 14.66297538114749344 ) ) ;
#21355=CARTESIAN_POINT ( 'NONE',  ( 8.700000000232593678, -29.57788259996195634, -26.81583080857759072 ) ) ;
#21358=( GEOMETRIC_REPRESENTATION_CONTEXT ( 3 ) GLOBAL_UNCERTAINTY_ASSIGNED_CONTEXT ( ( #29493 ) ) GLOBAL_UNIT_ASSIGNED_CONTEXT ( ( #11540, #16411, #26324 ) ) REPRESENTATION_CONTEXT ( 'NONE', 'WORKASPACE' ) );
#21381=CARTESIAN_POINT ( 'NONE',  ( -8.699999999640422033, -12.54233388092882784, -39.16320152032577795 ) ) ;
#21409=CARTESIAN_POINT ( 'NONE',  ( -7.999999999653043758, -13.95409160420028449, -37.06321646920958557 ) ) ;
#21421=ADVANCED_FACE ( 'NONE', ( #9699 ), #26231, .F. ) ;
#21437=DIRECTION ( 'NONE',  ( 1.000000000000000000, -1.843431230200084908E-12, 2.650498504963248473E-12 ) ) ;
#21438=ORIENTED_EDGE ( 'NONE', *, *, #15029, .T. ) ;
#21451=CYLINDRICAL_SURFACE ( 'NONE', #30048, 10.00000000000000178 ) ;
#21466=CARTESIAN_POINT ( 'NONE',  ( -8.699999999703425857, -29.80249410822303346, -29.47052640025896508 ) ) ;
#21474=CARTESIAN_POINT ( 'NONE',  ( 8.000000000250089727, -26.69041892760361279, -31.40984194550128805 ) ) ;
#21495=CARTESIAN_POINT ( 'NONE',  ( -7.999999999682144924, -15.00895261645561618, -33.21453337755221469 ) ) ;
#21497=CARTESIAN_POINT ( 'NONE',  ( 8.000000000264140709, -18.27877680372071723, -30.94409471150577318 ) ) ;
#21506=DIRECTION ( 'NONE',  ( -1.000000000000000000, 2.082932338114093583E-15, -6.768115529734696084E-12 ) ) ;
#21538=FACE_OUTER_BOUND ( 'NONE', #10494, .T. ) ;
#21580=CYLINDRICAL_SURFACE ( 'NONE', #17589, 2.500000000000001776 ) ;
#21601=VERTEX_POINT ( 'NONE', #3861 ) ;
#21611=CARTESIAN_POINT ( 'NONE',  ( -7.871622393891488656, -5.774860021632473028, -27.47894970137238957 ) ) ;
#21622=ADVANCED_FACE ( 'NONE', ( #20538, #13451 ), #23069, .T. ) ;
#21625=CARTESIAN_POINT ( 'NONE',  ( 8.000000000489755791, -29.44934466748925672, -30.17621036715362592 ) ) ;
#21630=EDGE_CURVE ( 'NONE', #61, #16882, #18333, .T. ) ;
#21638=B_SPLINE_CURVE_WITH_KNOTS ( 'NONE', 5,
 ( #19753, #9843, #29491, #5113, #29032, #10000, #4964, #19599, #10464 ),
 .UNSPECIFIED., .F., .F.,
 ( 6, 3, 6 ),
 ( 0.000000000000000000, 6.585924280900000483, 11.50063931930000116 ),
 .UNSPECIFIED. ) ;
#21645=ORIENTED_EDGE ( 'NONE', *, *, #13898, .F. ) ;
#21646=CARTESIAN_POINT ( 'NONE',  ( 8.000000000313141513, -13.45181286506001506, -44.64612647231290765 ) ) ;
#21712=CARTESIAN_POINT ( 'NONE',  ( -7.999999999650483140, -14.85786197181147372, -37.78376919401149792 ) ) ;
#21729=VECTOR ( 'NONE', #15964, 1000.000000000000000 ) ;
#21748=ORIENTED_EDGE ( 'NONE', *, *, #19458, .T. ) ;
#21771=LINE ( 'NONE', #17754, #16512 ) ;
#21787=DIRECTION ( 'NONE',  ( 7.759996349202911684E-13, 0.9341647027306021478, 0.3568421334038983650 ) ) ;
#21794=FACE_OUTER_BOUND ( 'NONE', #28517, .T. ) ;
#21802=CARTESIAN_POINT ( 'NONE',  ( 8.700000000242635423, -24.33830582822444200, -26.96109716006106893 ) ) ;
#21804=CARTESIAN_POINT ( 'NONE',  ( 8.700000000277906764, -15.94902145836247342, -35.53273252485295330 ) ) ;
#21807=AXIS2_PLACEMENT_3D ( 'NONE', #30293, #18331, #7150 ) ;
#21813=VECTOR ( 'NONE', #12914, 1000.000000000000000 ) ;
#21833=VECTOR ( 'NONE', #23179, 999.9999999999998863 ) ;
#21838=AXIS2_PLACEMENT_3D ( 'NONE', #11996, #28519, #23811 ) ;
#21839=AXIS2_PLACEMENT_3D ( 'NONE', #3890, #1539, #14812 ) ;
#21843=CARTESIAN_POINT ( 'NONE',  ( 8.700000000232995134, -27.30967745505199673, -25.39025505876632494 ) ) ;
#21846=CARTESIAN_POINT ( 'NONE',  ( 8.000000000248304488, -25.92947504235655032, -31.20249033167290165 ) ) ;
#21853=LINE ( 'NONE', #7055, #24007 ) ;
#21877=AXIS2_PLACEMENT_3D ( 'NONE', #16425, #1650, #2114 ) ;
#21887=CARTESIAN_POINT ( 'NONE',  ( -7.999999999728448330, -26.04217715522926824, -25.54542481146843613 ) ) ;
#21893=FACE_OUTER_BOUND ( 'NONE', #7113, .T. ) ;
#21916=B_SPLINE_CURVE_WITH_KNOTS ( 'NONE', 3,
 ( #27499, #12721, #27201, #22791, #5640, #19964 ),
 .UNSPECIFIED., .F., .F.,
 ( 4, 2, 4 ),
 ( 0.000000000000000000, 0.5000000000000000000, 1.000000000000000000 ),
 .UNSPECIFIED. ) ;
#21918=CARTESIAN_POINT ( 'NONE',  ( 7.999999999489469715, -115.5185322950121929, 21.06548255655121338 ) ) ;
#21927=CARTESIAN_POINT ( 'NONE',  ( -7.999999999683591767, -17.13607329101123611, -33.32374753170036286 ) ) ;
#21939=DIRECTION ( 'NONE',  ( 0.000000000000000000, -0.9128796883888953273, 0.4082287037029528887 ) ) ;
#21943=ORIENTED_EDGE ( 'NONE', *, *, #2908, .F. ) ;
#21959=ADVANCED_FACE ( 'NONE', ( #3043 ), #19580, .F. ) ;
#21960=EDGE_CURVE ( 'NONE', #2058, #22456, #15807, .T. ) ;
#21967=CARTESIAN_POINT ( 'NONE',  ( 8.700000000296066460, -14.31621543018684761, -40.15015555144486115 ) ) ;
#21971=CARTESIAN_POINT ( 'NONE',  ( -7.999999999681902452, -14.92844969907143771, -33.25053330396754347 ) ) ;
#21980=CARTESIAN_POINT ( 'NONE',  ( -7.999999999675157625, -13.69798478930254149, -34.44157303844319529 ) ) ;
#21998=CARTESIAN_POINT ( 'NONE',  ( 8.000000000250929943, -24.65281347431490033, -30.30937277425890386 ) ) ;
#22008=DIRECTION ( 'NONE',  ( 1.000000000000000000, -9.219999999999999084E-13, 4.710999999999999616E-12 ) ) ;
#22025=ADVANCED_FACE ( 'NONE', ( #3501 ), #29938, .F. ) ;
#22033=VERTEX_POINT ( 'NONE', #27573 ) ;
#22040=DIRECTION ( 'NONE',  ( -3.924189347185961537E-12, 0.4082287037029530552, 0.9128796883888952163 ) ) ;
#22079=DIRECTION ( 'NONE',  ( 7.759996349202911684E-13, 0.9341647027306021478, 0.3568421334038983650 ) ) ;
#22087=CARTESIAN_POINT ( 'NONE',  ( -8.699999999719173260, -29.89939565891263484, -27.53479725668291422 ) ) ;
#22117=DIRECTION ( 'NONE',  ( 1.000000000000000000, -1.843431230201421806E-12, 2.650498504952891752E-12 ) ) ;
#22120=DIRECTION ( 'NONE',  ( 3.582312748438143944E-12, 0.000000000000000000, -1.000000000000000000 ) ) ;
#22127=CARTESIAN_POINT ( 'NONE',  ( -8.700000000035505110, -116.0414483704498139, 19.89613934350620639 ) ) ;
#22130=CARTESIAN_POINT ( 'NONE',  ( -7.999999999674482609, -13.63932521616414029, -34.57331013702438582 ) ) ;
#22136=AXIS2_PLACEMENT_3D ( 'NONE', #136, #12536, #7510 ) ;
#22166=CARTESIAN_POINT ( 'NONE',  ( -7.999999999948583351, -112.9248453963972452, 6.301092398322726496 ) ) ;
#22196=FACE_OUTER_BOUND ( 'NONE', #18505, .T. ) ;
#22197=B_SPLINE_CURVE_WITH_KNOTS ( 'NONE', 5,
 ( #24034, #9553, #29054, #124, #24184, #23733, #11759, #440, #16781 ),
 .UNSPECIFIED., .F., .F.,
 ( 6, 3, 6 ),
 ( 0.000000000000000000, 0.6973066786029999964, 1.117931991990000151 ),
 .UNSPECIFIED. ) ;
#22198=CARTESIAN_POINT ( 'NONE',  ( 4.276011752470107119, -42.94729992904354532, -9.547410993441516780 ) ) ;
#22215=CARTESIAN_POINT ( 'NONE',  ( 7.760746006746995107, -115.2611165973680585, 21.64111469539790633 ) ) ;
#22218=ORIENTED_EDGE ( 'NONE', *, *, #23329, .T. ) ;
#22225=CARTESIAN_POINT ( 'NONE',  ( -7.999999999656285610, -17.88204346701441239, -37.14367873950658350 ) ) ;
#22258=ORIENTED_EDGE ( 'NONE', *, *, #24279, .T. ) ;
#22262=CARTESIAN_POINT ( 'NONE',  ( 1.057488903014505443E-10, -103.0613381315276484, 16.56805218638653798 ) ) ;
#22266=ORIENTED_EDGE ( 'NONE', *, *, #16369, .T. ) ;
#22268=PLANE ( 'NONE',  #27082 ) ;
#22282=CARTESIAN_POINT ( 'NONE',  ( -7.999999999678859552, -14.17437075046522210, -33.74882213760563587 ) ) ;
#22296=CARTESIAN_POINT ( 'NONE',  ( 8.700000000283306889, -21.59962967316020865, -40.40111538753404830 ) ) ;
#22357=B_SPLINE_CURVE_WITH_KNOTS ( 'NONE', 3,
 ( #19848, #20291, #29429, #13054, #8165, #5666 ),
 .UNSPECIFIED., .F., .F.,
 ( 4, 2, 4 ),
 ( 0.000000000000000000, 0.5000000000000000000, 1.000000000000000000 ),
 .UNSPECIFIED. ) ;
#22375=CARTESIAN_POINT ( 'NONE',  ( 7.734594132576882330, -115.2493501891094780, 21.66742669895628026 ) ) ;
#22378=AXIS2_PLACEMENT_3D ( 'NONE', #7275, #12142, #16702 ) ;
#22382=EDGE_LOOP ( 'NONE', ( #25676, #13420, #3908, #16177 ) ) ;
#22384=LINE ( 'NONE', #17635, #29222 ) ;
#22398=CARTESIAN_POINT ( 'NONE',  ( -7.999999999660042604, -18.28443193496838504, -36.42483736938474692 ) ) ;
#22406=CARTESIAN_POINT ( 'NONE',  ( -8.699999999683917906, -16.84112679184576677, -33.19732076807623145 ) ) ;
#22418=DIRECTION ( 'NONE',  ( 3.924189347185962345E-12, -0.4082287037029530552, -0.9128796883888953273 ) ) ;
#22431=EDGE_CURVE ( 'NONE', #13180, #3651, #22197, .T. ) ;
#22435=LINE ( 'NONE', #730, #17794 ) ;
#22440=CARTESIAN_POINT ( 'NONE',  ( 8.700000000244115128, -26.99999999999395328, -28.39999999994493862 ) ) ;
#22450=FACE_OUTER_BOUND ( 'NONE', #27897, .T. ) ;
#22456=VERTEX_POINT ( 'NONE', #26397 ) ;
#22470=LINE ( 'NONE', #617, #8614 ) ;
#22492=ORIENTED_EDGE ( 'NONE', *, *, #26690, .T. ) ;
#22503=DIRECTION ( 'NONE',  ( -7.764622278472185525E-13, -0.9341647027306024809, -0.3568421334038978099 ) ) ;
#22513=CYLINDRICAL_SURFACE ( 'NONE', #17241, 10.00000000000000533 ) ;
#22527=CARTESIAN_POINT ( 'NONE',  ( -7.999999999692643193, -25.56262797781471718, -31.06236252952192700 ) ) ;
#22571=ORIENTED_EDGE ( 'NONE', *, *, #22912, .F. ) ;
#22590=DIRECTION ( 'NONE',  ( -1.000000000000000000, 5.687697999151106851E-16, -6.771501495036750356E-12 ) ) ;
#22604=DIRECTION ( 'NONE',  ( -3.134067079931429195E-12, -0.3568421334038983650, 0.9341647027306021478 ) ) ;
#22606=CARTESIAN_POINT ( 'NONE',  ( 7.999999999820811780, -5.927567494231108292, -27.82043365066874685 ) ) ;
#22620=ADVANCED_FACE ( 'NONE', ( #12032 ), #12177, .F. ) ;
#22622=VERTEX_POINT ( 'NONE', #23695 ) ;
#22691=VECTOR ( 'NONE', #4903, 1000.000000000000000 ) ;
#22708=ORIENTED_EDGE ( 'NONE', *, *, #5927, .T. ) ;
#22726=CARTESIAN_POINT ( 'NONE',  ( 8.000000000285856672, -13.61361098174325868, -34.64062768040190576 ) ) ;
#22768=CARTESIAN_POINT ( 'NONE',  ( -8.699999999718064814, -24.05685110469877230, -27.69790561507143778 ) ) ;
#22774=FACE_OUTER_BOUND ( 'NONE', #10742, .T. ) ;
#22783=EDGE_CURVE ( 'NONE', #11991, #22622, #30430, .T. ) ;
#22791=CARTESIAN_POINT ( 'NONE',  ( -8.699999999678249551, -14.35760254608830522, -33.57685301057431815 ) ) ;
#22826=ORIENTED_EDGE ( 'NONE', *, *, #26550, .T. ) ;
#22839=VERTEX_POINT ( 'NONE', #20665 ) ;
#22845=CARTESIAN_POINT ( 'NONE',  ( -4.276011752185619130, -51.11187400311629858, -27.80500476125005704 ) ) ;
#22846=CARTESIAN_POINT ( 'NONE',  ( -8.699999999648646565, -16.67007951101791363, -37.94887063592300791 ) ) ;
#22860=ADVANCED_FACE ( 'NONE', ( #2253 ), #5065, .F. ) ;
#22877=B_SPLINE_CURVE_WITH_KNOTS ( 'NONE', 3,
 ( #26250, #19474, #21843, #9714, #26865, #14296 ),
 .UNSPECIFIED., .F., .F.,
 ( 4, 2, 4 ),
 ( 0.000000000000000000, 0.5000000000000000000, 1.000000000000000000 ),
 .UNSPECIFIED. ) ;
#22890=DIRECTION ( 'NONE',  ( -6.181333986565961785E-12, 0.4082287037029530552, 0.9128796883888953273 ) ) ;
#22896=ORIENTED_EDGE ( 'NONE', *, *, #23830, .T. ) ;
#22903=CARTESIAN_POINT ( 'NONE',  ( 8.000000000467634820, -18.45959768780296173, -35.96628083219813021 ) ) ;
#22912=EDGE_CURVE ( 'NONE', #9163, #14716, #16865, .T. ) ;
#22918=ADVANCED_FACE ( 'NONE', ( #4598 ), #21135, .F. ) ;
#22921=CARTESIAN_POINT ( 'NONE',  ( -8.699999999731478084, -27.30911655878985300, -25.39023929165498572 ) ) ;
#22923=VERTEX_POINT ( 'NONE', #26319 ) ;
#22936=CYLINDRICAL_SURFACE ( 'NONE', #13290, 1.700000000000000178 ) ;
#22940=CARTESIAN_POINT ( 'NONE',  ( 8.700000000248305554, -25.92947359976189503, -31.20249410819006286 ) ) ;
#22975=DIRECTION ( 'NONE',  ( -3.112440860597585673E-12, -0.3322662713817149949, 0.9431856258987901809 ) ) ;
#22977=CARTESIAN_POINT ( 'NONE',  ( -7.999999999636759895, -22.42568788229198873, -40.05522481832764470 ) ) ;
#23040=VERTEX_POINT ( 'NONE', #12604 ) ;
#23041=CARTESIAN_POINT ( 'NONE',  ( -8.699999999651764071, -17.54044037066235617, -37.48861203924890617 ) ) ;
#23051=FACE_BOUND ( 'NONE', #20832, .T. ) ;
#23066=FACE_OUTER_BOUND ( 'NONE', #4136, .T. ) ;
#23069=PLANE ( 'NONE',  #27348 ) ;
#23076=CARTESIAN_POINT ( 'NONE',  ( 8.000000000281330514, -5.981227587277713198, -27.94042817480428198 ) ) ;
#23079=VERTEX_POINT ( 'NONE', #27086 ) ;
#23086=VERTEX_POINT ( 'NONE', #5829 ) ;
#23089=DIRECTION ( 'NONE',  ( 1.000000000000000000, -1.843431230201421806E-12, 2.650498504952891752E-12 ) ) ;
#23091=CYLINDRICAL_SURFACE ( 'NONE', #1772, 2.500000000000002220 ) ;
#23108=AXIS2_PLACEMENT_3D ( 'NONE', #22845, #5537, #19875 ) ;
#23110=CARTESIAN_POINT ( 'NONE',  ( -6.999999999263968320, -5.430118837242332575, -26.70804059545048759 ) ) ;
#23117=EDGE_CURVE ( 'NONE', #9868, #15244, #27235, .T. ) ;
#23125=EDGE_CURVE ( 'NONE', #17663, #27730, #28874, .T. ) ;
#23129=CARTESIAN_POINT ( 'NONE',  ( 8.000000000284819279, -13.66682223737133128, -36.55330428412179344 ) ) ;
#23144=CARTESIAN_POINT ( 'NONE',  ( 8.700000000236814302, -30.00974564182223503, -28.70967732804903605 ) ) ;
#23146=VERTEX_POINT ( 'NONE', #5214 ) ;
#23161=CARTESIAN_POINT ( 'NONE',  ( 8.000000000645886900, -15.87764099349055158, -32.96702544412416813 ) ) ;
#23177=CARTESIAN_POINT ( 'NONE',  ( 8.000000000278095769, -14.92844969908619035, -33.25053330389217621 ) ) ;
#23179=DIRECTION ( 'NONE',  ( 2.764840495839172918E-12, 0.9128796883888953273, -0.4082287037029531107 ) ) ;
#23185=B_SPLINE_CURVE_WITH_KNOTS ( 'NONE', 5,
 ( #12112, #19361, #7393, #26595, #14644, #2673, #12270, #21887, #7693, #19668, #5343, #5180 ),
 .UNSPECIFIED., .F., .F.,
 ( 6, 3, 3, 6 ),
 ( 3.339306057039999942, 4.810258469309999896, 6.613963844750000654, 6.678484288699999993 ),
 .UNSPECIFIED. ) ;
#23195=CARTESIAN_POINT ( 'NONE',  ( -8.699999999654988159, -17.99042170907872418, -37.01252660134724692 ) ) ;
#23200=VECTOR ( 'NONE', #27073, 999.9999999999998863 ) ;
#23205=ORIENTED_EDGE ( 'NONE', *, *, #5927, .F. ) ;
#23238=VECTOR ( 'NONE', #17154, 1000.000000000000000 ) ;
#23240=CARTESIAN_POINT ( 'NONE',  ( -8.699999999669005391, -18.23122067931867107, -34.51216076567753532 ) ) ;
#23244=CARTESIAN_POINT ( 'NONE',  ( 8.700000000245456278, -28.58416947897984173, -30.97788247129344086 ) ) ;
#23266=ADVANCED_FACE ( 'NONE', ( #4096 ), #13065, .F. ) ;
#23268=ORIENTED_EDGE ( 'NONE', *, *, #28811, .T. ) ;
#23269=PRODUCT_CONTEXT ( 'NONE', #3128, 'mechanical' ) ;
#23276=CARTESIAN_POINT ( 'NONE',  ( -8.699999998949005331, -18.23122067931867107, -34.51216076567753532 ) ) ;
#23293=CARTESIAN_POINT ( 'NONE',  ( 8.700000000290035729, -14.46884615155692977, -37.57385308047970796 ) ) ;
#23294=CARTESIAN_POINT ( 'NONE',  ( 8.700000000235821318, -29.73863906516063693, -27.17531388883607590 ) ) ;
#23328=STYLED_ITEM ( 'NONE', ( #8783 ), #438 ) ;
#23329=EDGE_CURVE ( 'NONE', #30101, #8184, #3337, .T. ) ;
#23337=LINE ( 'NONE', #6639, #5757 ) ;
#23341=VERTEX_POINT ( 'NONE', #30844 ) ;
#23344=CARTESIAN_POINT ( 'NONE',  ( -5.712231154917421249E-11, -114.8328013978253495, 22.59891173985517199 ) ) ;
#23359=LINE ( 'NONE', #1638, #15476 ) ;
#23388=EDGE_CURVE ( 'NONE', #21601, #27055, #13162, .T. ) ;
#23389=ORIENTED_EDGE ( 'NONE', *, *, #28054, .F. ) ;
#23397=ORIENTED_EDGE ( 'NONE', *, *, #7072, .F. ) ;
#23418=PLANE ( 'NONE',  #2105 ) ;
#23420=CARTESIAN_POINT ( 'NONE',  ( 8.700000000247927190, -27.47597782793287990, -31.38791861936106287 ) ) ;
#23433=ADVANCED_FACE ( 'NONE', ( #16005 ), #8759, .F. ) ;
#23440=FILL_AREA_STYLE_COLOUR ( '', #5720 ) ;
#23455=CARTESIAN_POINT ( 'NONE',  ( -8.000000000030556890, -116.5561065465021784, 18.74526241810166027 ) ) ;
#23469=VERTEX_POINT ( 'NONE', #15854 ) ;
#23499=ORIENTED_EDGE ( 'NONE', *, *, #4048, .T. ) ;
#23512=( NAMED_UNIT ( * ) SI_UNIT ( $, .STERADIAN. ) SOLID_ANGLE_UNIT ( ) );
#23516=EDGE_CURVE ( 'NONE', #24719, #10063, #6864, .T. ) ;
#23532=CARTESIAN_POINT ( 'NONE',  ( -8.699999999683917906, -16.84112679184576677, -33.19732076807623145 ) ) ;
#23577=CARTESIAN_POINT ( 'NONE',  ( 8.700000000249431764, -26.69088343938642538, -31.40976070819087695 ) ) ;
#23618=CARTESIAN_POINT ( 'NONE',  ( 8.700000000249179521, -24.10030203291533368, -29.26452672280898781 ) ) ;
#23624=ORIENTED_EDGE ( 'NONE', *, *, #24279, .F. ) ;
#23625=ORIENTED_EDGE ( 'NONE', *, *, #27192, .T. ) ;
#23647=VECTOR ( 'NONE', #8865, 1000.000000000000227 ) ;
#23652=ORIENTED_EDGE ( 'NONE', *, *, #26550, .F. ) ;
#23656=CARTESIAN_POINT ( 'NONE',  ( 8.700000000273238498, -16.53478705811768990, -33.08035312245812776 ) ) ;
#23660=DIRECTION ( 'NONE',  ( 1.000000000000000000, -1.843431230200084908E-12, 2.650498504963248473E-12 ) ) ;
#23665=ORIENTED_EDGE ( 'NONE', *, *, #30739, .F. ) ;
#23668=B_SPLINE_CURVE_WITH_KNOTS ( 'NONE', 5,
 ( #27435, #29328, #19901, #3207, #714, #15023, #29483, #3356, #7922 ),
 .UNSPECIFIED., .F., .F.,
 ( 6, 3, 6 ),
 ( 0.000000000000000000, 6.585791975970000323, 10.75845894650000112 ),
 .UNSPECIFIED. ) ;
#23682=ORIENTED_EDGE ( 'NONE', *, *, #6232, .F. ) ;
#23693=CARTESIAN_POINT ( 'NONE',  ( -7.999999999668092165, -18.32608219842778752, -34.72428978364464314 ) ) ;
#23695=CARTESIAN_POINT ( 'NONE',  ( -6.999999999597122269, -114.8328013979413527, 22.59891173954833477 ) ) ;
#23707=ORIENTED_EDGE ( 'NONE', *, *, #17169, .T. ) ;
#23711=DIRECTION ( 'NONE',  ( -1.000000000000000000, 1.843431230205392516E-12, -2.650498504954667282E-12 ) ) ;
#23721=CARTESIAN_POINT ( 'NONE',  ( 8.700000000235821318, -29.73863906516063693, -27.17531388883607590 ) ) ;
#23731=CARTESIAN_POINT ( 'NONE',  ( -7.999999999728899525, -28.83899161331666150, -25.99720916226845091 ) ) ;
#23733=CARTESIAN_POINT ( 'NONE',  ( 7.572771919626319459, -115.1908526478854071, 21.79823870879123504 ) ) ;
#23739=ORIENTED_EDGE ( 'NONE', *, *, #10797, .F. ) ;
#23744=ORIENTED_EDGE ( 'NONE', *, *, #22783, .F. ) ;
#23745=DIRECTION ( 'NONE',  ( 1.000000000000000000, -1.843431230198065424E-12, 2.650498504953516580E-12 ) ) ;
#23746=CARTESIAN_POINT ( 'NONE',  ( -8.699999999660271044, -9.763725516012462080, -36.23155182226569337 ) ) ;
#23754=VERTEX_POINT ( 'NONE', #24327 ) ;
#23765=DIRECTION ( 'NONE',  ( -1.000000000000000000, 5.687697913155423197E-16, -6.771501495041734442E-12 ) ) ;
#23778=ORIENTED_EDGE ( 'NONE', *, *, #6445, .T. ) ;
#23811=DIRECTION ( 'NONE',  ( 3.112440860597585673E-12, 0.3322662713817149949, -0.9431856258987901809 ) ) ;
#23815=ORIENTED_EDGE ( 'NONE', *, *, #30470, .T. ) ;
#23823=EDGE_CURVE ( 'NONE', #23079, #9796, #17087, .T. ) ;
#23830=EDGE_CURVE ( 'NONE', #30177, #16921, #435, .T. ) ;
#23846=CARTESIAN_POINT ( 'NONE',  ( 8.699999999567717524, -16.96959321761985606, -37.81493174582519146 ) ) ;
#23855=PLANE ( 'NONE',  #11949 ) ;
#23869=CARTESIAN_POINT ( 'NONE',  ( 8.700000000296048697, -11.00364569656339775, -37.83911830543074473 ) ) ;
#23872=CARTESIAN_POINT ( 'NONE',  ( 8.700000000241731257, -29.44972865398396067, -30.17591950688898095 ) ) ;
#23879=CARTESIAN_POINT ( 'NONE',  ( -8.349999999348669988, -5.981227587280896429, -27.94042817487314423 ) ) ;
#23904=ORIENTED_EDGE ( 'NONE', *, *, #14092, .F. ) ;
#23905=VECTOR ( 'NONE', #227, 1000.000000000000000 ) ;
#23907=CARTESIAN_POINT ( 'NONE',  ( -8.699999999643161175, -12.00129099599161897, -38.75807114290937250 ) ) ;
#23923=DIRECTION ( 'NONE',  ( -3.133604487004501508E-12, -0.3568421334038989756, 0.9341647027306019258 ) ) ;
#23924=CARTESIAN_POINT ( 'NONE',  ( 8.000000000276081380, -16.84112630282697154, -33.19732204816383359 ) ) ;
#23925=CARTESIAN_POINT ( 'NONE',  ( 8.699999999959866059, -117.3672015275926697, 16.33620430255450628 ) ) ;
#23948=ADVANCED_FACE ( 'NONE', ( #5746 ), #27610, .F. ) ;
#23955=CARTESIAN_POINT ( 'NONE',  ( -8.699999999785086757, -66.94093258035375982, -17.28188441703444411 ) ) ;
#23964=CARTESIAN_POINT ( 'NONE',  ( -8.700000000030557956, -116.5561065468281186, 18.74526241736806043 ) ) ;
#23972=ORIENTED_EDGE ( 'NONE', *, *, #27821, .F. ) ;
#23973=FACE_OUTER_BOUND ( 'NONE', #25665, .T. ) ;
#23975=CARTESIAN_POINT ( 'NONE',  ( -7.999999999671499218, -17.87438019985146553, -33.91263442688144636 ) ) ;
#23991=CARTESIAN_POINT ( 'NONE',  ( 8.000000000236575204, -29.80249033211431708, -29.47052495773638370 ) ) ;
#24007=VECTOR ( 'NONE', #14146, 999.9999999999998863 ) ;
#24015=DIRECTION ( 'NONE',  ( 0.000000000000000000, -0.9128796883888953273, 0.4082287037029528332 ) ) ;
#24018=CARTESIAN_POINT ( 'NONE',  ( -7.999999999684019869, -16.03708229645564742, -33.01798262065937450 ) ) ;
#24027=CARTESIAN_POINT ( 'NONE',  ( -8.699999999729206124, -25.09057560198417747, -26.05270539051472767 ) ) ;
#24034=CARTESIAN_POINT ( 'NONE',  ( 6.999999999945624829, -115.1185614904238577, 21.95989595801592031 ) ) ;
#24036=ADVANCED_FACE ( 'NONE', ( #23066 ), #1509, .F. ) ;
#24039=SHAPE_REPRESENTATION ( 'Moving Handle', ( #17722 ), #9278 ) ;
#24048=ORIENTED_EDGE ( 'NONE', *, *, #14444, .F. ) ;
#24050=B_SPLINE_CURVE_WITH_KNOTS ( 'NONE', 3,
 ( #18307, #17979, #28214, #27590, #16255, #6351, #15629, #25875, #25239, #25404 ),
 .UNSPECIFIED., .F., .F.,
 ( 4, 2, 2, 2, 4 ),
 ( 0.000000000000000000, 0.2500000000000000000, 0.5000000000000000000, 0.7500000000000000000, 1.000000000000000000 ),
 .UNSPECIFIED. ) ;
#24054=EDGE_CURVE ( 'NONE', #28713, #28185, #2576, .T. ) ;
#24073=VECTOR ( 'NONE', #11632, 999.9999999999998863 ) ;
#24082=ORIENTED_EDGE ( 'NONE', *, *, #16916, .F. ) ;
#24102=CARTESIAN_POINT ( 'NONE',  ( 8.699999999569731912, -15.05691612486679176, -37.86814428171000912 ) ) ;
#24112=ADVANCED_FACE ( 'NONE', ( #26047, #14087 ), #13929, .F. ) ;
#24115=VECTOR ( 'NONE', #3801, 1000.000000000000000 ) ;
#24125=PLANE ( 'NONE',  #24796 ) ;
#24134=B_SPLINE_CURVE_WITH_KNOTS ( 'NONE', 4,
 ( #28146, #16185, #6432, #29879, #23129 ),
 .UNSPECIFIED., .F., .F.,
 ( 5, 5 ),
 ( -0.9817477042479999527, 0.9817477042479999527 ),
 .UNSPECIFIED. ) ;
#24136=CARTESIAN_POINT ( 'NONE',  ( -7.999999999650188265, -15.90960369693041088, -38.05208140759208391 ) ) ;
#24155=DIRECTION ( 'NONE',  ( 1.000000000000000000, -9.219999999999999084E-13, 4.710999999999999616E-12 ) ) ;
#24163=CYLINDRICAL_SURFACE ( 'NONE', #27806, 2.500000000000000888 ) ;
#24165=CARTESIAN_POINT ( 'NONE',  ( 8.699999999551790708, -9.149979919791583427, -35.02638174844071983 ) ) ;
#24169=CARTESIAN_POINT ( 'NONE',  ( 8.700000000290671665, -15.69142432425455347, -38.04086644837175157 ) ) ;
#24184=CARTESIAN_POINT ( 'NONE',  ( 7.439629836415988962, -115.1565018356284327, 21.87505388250205129 ) ) ;
#24194=ORIENTED_EDGE ( 'NONE', *, *, #3586, .T. ) ;
#24196=( LENGTH_UNIT ( ) NAMED_UNIT ( * ) SI_UNIT ( .MILLI., .METRE. ) );
#24204=VERTEX_POINT ( 'NONE', #4943 ) ;
#24256=CARTESIAN_POINT ( 'NONE',  ( -7.999999999718343524, -24.19750589173343869, -27.32947359979155166 ) ) ;
#24279=EDGE_CURVE ( 'NONE', #6080, #10911, #14948, .T. ) ;
#24282=CARTESIAN_POINT ( 'NONE',  ( -7.999999999650268201, -15.05691661382650537, -37.86814300153927348 ) ) ;
#24316=CYLINDRICAL_SURFACE ( 'NONE', #10790, 10.00000000000000178 ) ;
#24319=VECTOR ( 'NONE', #17545, 1000.000000000000000 ) ;
#24327=CARTESIAN_POINT ( 'NONE',  ( -8.699999999718668775, -5.981227587262315737, -27.94042817488295682 ) ) ;
#24331=AXIS2_PLACEMENT_3D ( 'NONE', #1869, #23745, #20914 ) ;
#24342=ORIENTED_EDGE ( 'NONE', *, *, #4891, .F. ) ;
#24347=VECTOR ( 'NONE', #11257, 1000.000000000000114 ) ;
#24372=AXIS2_PLACEMENT_3D ( 'NONE', #17362, #24760, #5254 ) ;
#24410=CARTESIAN_POINT ( 'NONE',  ( -7.999999999688209407, -9.149979919817011975, -35.02638174861068165 ) ) ;
#24442=EDGE_CURVE ( 'NONE', #2785, #18386, #23337, .T. ) ;
#24447=CARTESIAN_POINT ( 'NONE',  ( 8.349999999921791982, -9.149979919791261906, -35.02638174844237540 ) ) ;
#24451=CARTESIAN_POINT ( 'NONE',  ( 8.000000000473534101, -13.78877417416307871, -34.18207016520864983 ) ) ;
#24457=CARTESIAN_POINT ( 'NONE',  ( -8.699999999671032214, -18.09762814832684796, -34.21342158600526062 ) ) ;
#24492=CARTESIAN_POINT ( 'NONE',  ( -7.999999999729964451, -28.19367756375590872, -25.64455236481611777 ) ) ;
#24510=VECTOR ( 'NONE', #20278, 1000.000000000000000 ) ;
#24527=CARTESIAN_POINT ( 'NONE',  ( -7.999999999971132425, -116.4789120197461187, 10.39182877040068931 ) ) ;
#24537=EDGE_CURVE ( 'NONE', #6463, #3666, #13572, .T. ) ;
#24557=EDGE_LOOP ( 'NONE', ( #4306, #8300, #27028, #24614 ) ) ;
#24582=ORIENTED_EDGE ( 'NONE', *, *, #18072, .F. ) ;
#24592=DIRECTION ( 'NONE',  ( -6.386904893851405129E-12, -0.3322662713817149949, 0.9431856258987901809 ) ) ;
#24607=CARTESIAN_POINT ( 'NONE',  ( -7.999999999721752353, -29.89895010230364392, -27.53380090445090289 ) ) ;
#24614=ORIENTED_EDGE ( 'NONE', *, *, #30256, .T. ) ;
#24625=CARTESIAN_POINT ( 'NONE',  ( 8.700000000229927366, -28.07050130669910715, -25.59757157921452020 ) ) ;
#24632=CARTESIAN_POINT ( 'NONE',  ( 8.700000000244115128, -26.99999999999395328, -28.39999999994493862 ) ) ;
#24643=CARTESIAN_POINT ( 'NONE',  ( -7.999999999677900320, -14.01599944959732369, -33.92178631050306592 ) ) ;
#24658=ORIENTED_EDGE ( 'NONE', *, *, #4381, .F. ) ;
#24687=CARTESIAN_POINT ( 'NONE',  ( -8.699999998994179862, -29.73863906514459643, -27.17531388891805477 ) ) ;
#24693=ORIENTED_EDGE ( 'NONE', *, *, #16916, .T. ) ;
#24712=LINE ( 'NONE', #8164, #23200 ) ;
#24715=VECTOR ( 'NONE', #29895, 1000.000000000000000 ) ;
#24719=VERTEX_POINT ( 'NONE', #19994 ) ;
#24726=ORIENTED_EDGE ( 'NONE', *, *, #20654, .F. ) ;
#24738=CARTESIAN_POINT ( 'NONE',  ( 4.276011752470107119, -102.7755780389287281, 17.20706796827408169 ) ) ;
#24760=DIRECTION ( 'NONE',  ( -1.000000000000000000, 5.687698019341907056E-16, -6.771501495046482653E-12 ) ) ;
#24791=CARTESIAN_POINT ( 'NONE',  ( 8.000000000645206555, -18.51472853907661786, -35.46135205997079254 ) ) ;
#24796=AXIS2_PLACEMENT_3D ( 'NONE', #14843, #17342, #26785 ) ;
#24798=CARTESIAN_POINT ( 'NONE',  ( -7.999999999676562723, -13.83675952871606007, -34.17038780918873897 ) ) ;
#24801=ORIENTED_EDGE ( 'NONE', *, *, #23516, .T. ) ;
#24804=CARTESIAN_POINT ( 'NONE',  ( -7.999999999650326821, -14.98959907041461292, -37.84242876710612791 ) ) ;
#24836=CARTESIAN_POINT ( 'NONE',  ( 8.700000000277906764, -15.94902145836247342, -35.53273252485295330 ) ) ;
#24850=VERTEX_POINT ( 'NONE', #13532 ) ;
#24861=CARTESIAN_POINT ( 'NONE',  ( 8.000000000470132377, -15.51547315099485935, -38.04330875429763381 ) ) ;
#24889=VECTOR ( 'NONE', #15278, 1000.000000000000000 ) ;
#24895=EDGE_CURVE ( 'NONE', #14716, #19543, #8920, .T. ) ;
#24900=CYLINDRICAL_SURFACE ( 'NONE', #28107, 3.000000000000002220 ) ;
#24908=LINE ( 'NONE', #15000, #16018 ) ;
#24928=ADVANCED_FACE ( 'NONE', ( #13373 ), #2050, .T. ) ;
#24929=CARTESIAN_POINT ( 'NONE',  ( -7.999999999718343524, -24.19750589173343869, -27.32947359979155166 ) ) ;
#24956=DIRECTION ( 'NONE',  ( 1.000000000000000000, -1.843431230208684274E-12, 2.650498504958264790E-12 ) ) ;
#24974=CARTESIAN_POINT ( 'NONE',  ( -8.699999999710087195, -24.01208115640663010, -28.87640755789744063 ) ) ;
#24984=DIRECTION ( 'NONE',  ( -2.764840495839172514E-12, -0.9128796883888952163, 0.4082287037029530552 ) ) ;
#24988=ORIENTED_EDGE ( 'NONE', *, *, #13486, .F. ) ;
#24995=VERTEX_POINT ( 'NONE', #12098 ) ;
#25005=CARTESIAN_POINT ( 'NONE',  ( 7.999999999974046538, -116.8591659214849159, 11.34031266730467813 ) ) ;
#25026=CARTESIAN_POINT ( 'NONE',  ( -8.699999999660121830, -13.53288334731636233, -36.25379057756155277 ) ) ;
#25040=VECTOR ( 'NONE', #5190, 1000.000000000000000 ) ;
#25045=CARTESIAN_POINT ( 'NONE',  ( -7.999999999652283478, -16.96959321758620476, -37.81493174591201978 ) ) ;
#25072=VECTOR ( 'NONE', #21506, 1000.000000000000000 ) ;
#25074=ORIENTED_EDGE ( 'NONE', *, *, #7347, .T. ) ;
#25123=EDGE_CURVE ( 'NONE', #26249, #12816, #2515, .T. ) ;
#25145=ORIENTED_EDGE ( 'NONE', *, *, #14635, .T. ) ;
#25150=B_SPLINE_CURVE_WITH_KNOTS ( 'NONE', 3,
 ( #10419, #20011, #26784, #15287, #10112, #2866 ),
 .UNSPECIFIED., .F., .F.,
 ( 4, 2, 4 ),
 ( 0.000000000000000000, 0.5000000000000000000, 1.000000000000000000 ),
 .UNSPECIFIED. ) ;
#25167=CARTESIAN_POINT ( 'NONE',  ( 8.000000000654496901, -17.81372394443670615, -37.29648778942958387 ) ) ;
#25196=CARTESIAN_POINT ( 'NONE',  ( 8.699999999550994900, -18.23122067933471158, -34.51216076559557422 ) ) ;
#25212=EDGE_CURVE ( 'NONE', #6605, #22456, #2969, .T. ) ;
#25225=EDGE_CURVE ( 'NONE', #9796, #27055, #25932, .T. ) ;
#25236=ORIENTED_EDGE ( 'NONE', *, *, #9471, .T. ) ;
#25238=EDGE_CURVE ( 'NONE', #7991, #23341, #27650, .T. ) ;
#25239=CARTESIAN_POINT ( 'NONE',  ( -8.699999999633703851, -22.22846246279628346, -40.15612242420909439 ) ) ;
#25246=LINE ( 'NONE', #29957, #23647 ) ;
#25263=ORIENTED_EDGE ( 'NONE', *, *, #13506, .F. ) ;
#25288=ORIENTED_EDGE ( 'NONE', *, *, #2689, .T. ) ;
#25294=DIRECTION ( 'NONE',  ( -0.7071067811898219535, 0.2886612846638016983, 0.6455034180634624530 ) ) ;
#25316=ORIENTED_EDGE ( 'NONE', *, *, #28426, .T. ) ;
#25343=ORIENTED_EDGE ( 'NONE', *, *, #13369, .T. ) ;
#25348=DIRECTION ( 'NONE',  ( -2.764840495839172918E-12, -0.9128796883888953273, 0.4082287037029531107 ) ) ;
#25389=VECTOR ( 'NONE', #23660, 1000.000000000000000 ) ;
#25398=ORIENTED_EDGE ( 'NONE', *, *, #6885, .F. ) ;
#25404=CARTESIAN_POINT ( 'NONE',  ( -8.699999999638116321, -22.83323352287542463, -39.84673049988318638 ) ) ;
#25425=DIRECTION ( 'NONE',  ( -3.924189347185962345E-12, 0.4082287037029530552, 0.9128796883888953273 ) ) ;
#25442=CARTESIAN_POINT ( 'NONE',  ( -8.699999999737658030, -25.77531388886905006, -25.66136093486021608 ) ) ;
#25448=CARTESIAN_POINT ( 'NONE',  ( -8.699999999663262429, -18.45724128289285204, -35.79059583716231430 ) ) ;
#25460=ADVANCED_FACE ( 'NONE', ( #19150 ), #28740, .F. ) ;
#25470=ORIENTED_EDGE ( 'NONE', *, *, #19444, .F. ) ;
#25494=CARTESIAN_POINT ( 'NONE',  ( -7.999999999627648961, -16.75972747693622722, -40.88001126969393084 ) ) ;
#25499=CARTESIAN_POINT ( 'NONE',  ( 8.700000000237981368, -29.94290473664190699, -29.10277714274672434 ) ) ;
#25504=EDGE_LOOP ( 'NONE', ( #6877, #30661, #5266, #15772 ) ) ;
#25518=DIRECTION ( 'NONE',  ( -1.000000000000000000, 5.687697999151106851E-16, -6.771501495036750356E-12 ) ) ;
#25519=CARTESIAN_POINT ( 'NONE',  ( 8.000000000276081380, -16.84112630282697154, -33.19732204816383359 ) ) ;
#25543=ORIENTED_EDGE ( 'NONE', *, *, #4274, .F. ) ;
#25549=EDGE_LOOP ( 'NONE', ( #28056, #23665, #6928, #1481 ) ) ;
#25554=PRESENTATION_STYLE_ASSIGNMENT (( #28371 ) ) ;
#25555=VERTEX_POINT ( 'NONE', #11840 ) ;
#25603=DIRECTION ( 'NONE',  ( -3.924189347185962345E-12, 0.4082287037029530552, 0.9128796883888952163 ) ) ;
#25605=CARTESIAN_POINT ( 'NONE',  ( 8.000000000331638716, -14.95611408989132052, -40.37595097046627046 ) ) ;
#25617=DIRECTION ( 'NONE',  ( -6.325958275728752229E-12, -0.3568421334038983650, 0.9341647027306021478 ) ) ;
#25632=ORIENTED_EDGE ( 'NONE', *, *, #9967, .T. ) ;
#25642=CARTESIAN_POINT ( 'NONE',  ( -8.699999999985950083, -116.8589940772574920, 11.34037319969351643 ) ) ;
#25656=CARTESIAN_POINT ( 'NONE',  ( -7.999999999949311658, -29.44934466747404755, -30.17621036722960426 ) ) ;
#25665=EDGE_LOOP ( 'NONE', ( #23652, #12525, #1653, #1724 ) ) ;
#25676=ORIENTED_EDGE ( 'NONE', *, *, #16171, .F. ) ;
#25693=DIRECTION ( 'NONE',  ( 2.764840495839172918E-12, 0.9128796883888953273, -0.4082287037029530552 ) ) ;
#25722=CARTESIAN_POINT ( 'NONE',  ( 8.000000000361213282, -29.94262568628330357, -29.10368077924198715 ) ) ;
#25732=B_SPLINE_CURVE_WITH_KNOTS ( 'NONE', 3,
 ( #23532, #14082, #27929, #30610, #20855, #4168 ),
 .UNSPECIFIED., .F., .F.,
 ( 4, 2, 4 ),
 ( 0.000000000000000000, 0.5000000000000000000, 1.000000000000000000 ),
 .UNSPECIFIED. ) ;
#25741=CARTESIAN_POINT ( 'NONE',  ( -8.699999999985950083, -116.8589940772574920, 11.34037319969351643 ) ) ;
#25771=CARTESIAN_POINT ( 'NONE',  ( -8.000000000457589522, -24.26136093481186862, -29.62468611113247263 ) ) ;
#25784=DIRECTION ( 'NONE',  ( 1.000000000000000000, -1.953112501701599149E-12, 2.703609717165946368E-12 ) ) ;
#25794=DIRECTION ( 'NONE',  ( 3.924189347185962345E-12, -0.4082287037029530552, -0.9128796883888953273 ) ) ;
#25875=CARTESIAN_POINT ( 'NONE',  ( -8.699999999632044734, -21.59934857482445381, -40.40126712747085236 ) ) ;
#25879=CARTESIAN_POINT ( 'NONE',  ( 8.000000000235820252, -29.73863906515999389, -27.17531388883937993 ) ) ;
#25906=ORIENTED_EDGE ( 'NONE', *, *, #496, .T. ) ;
#25909=ORIENTED_EDGE ( 'NONE', *, *, #8216, .T. ) ;
#25915=DIRECTION ( 'NONE',  ( 2.764802276011834339E-12, 0.9128796883888953273, -0.4082287037029531107 ) ) ;
#25932=LINE ( 'NONE', #23110, #14832 ) ;
#25970=B_SPLINE_CURVE_WITH_KNOTS ( 'NONE', 3,
 ( #14589, #6752, #4243, #11014, #8957, #20762 ),
 .UNSPECIFIED., .F., .F.,
 ( 4, 2, 4 ),
 ( 0.000000000000000000, 0.5000000000000000000, 1.000000000000000000 ),
 .UNSPECIFIED. ) ;
#26017=EDGE_LOOP ( 'NONE', ( #30179, #24658, #10914, #17027 ) ) ;
#26027=CARTESIAN_POINT ( 'NONE',  ( 6.999999999949548801, -115.5267901941268178, 21.04701626962702576 ) ) ;
#26047=FACE_BOUND ( 'NONE', #21032, .T. ) ;
#26086=CARTESIAN_POINT ( 'NONE',  ( -7.999999999725509348, -29.60008687027021423, -26.86548392513261518 ) ) ;
#26106=CARTESIAN_POINT ( 'NONE',  ( 8.700000000279958456, -18.28438020625039329, -36.42481760783426381 ) ) ;
#26122=CARTESIAN_POINT ( 'NONE',  ( -8.000000000002907896, -107.4273096626132116, 14.66297538107212262 ) ) ;
#26153=CARTESIAN_POINT ( 'NONE',  ( -5.437537900614403780E-11, -115.1185614904174059, 21.95989595798294758 ) ) ;
#26167=EDGE_LOOP ( 'NONE', ( #8367, #26473, #30108, #20124 ) ) ;
#26171=DIRECTION ( 'NONE',  ( 1.000000000000000000, -1.843431230206220100E-12, 2.650498504954374861E-12 ) ) ;
#26183=AXIS2_PLACEMENT_3D ( 'NONE', #1546, #16161, #18200 ) ;
#26199=CARTESIAN_POINT ( 'NONE',  ( -7.999999999666060901, -18.44015901058016738, -35.17782714789814946 ) ) ;
#26200=B_SPLINE_CURVE_WITH_KNOTS ( 'NONE', 3,
 ( #12190, #26670, #9997, #29028, #21802, #14720 ),
 .UNSPECIFIED., .F., .F.,
 ( 4, 2, 4 ),
 ( 0.000000000000000000, 0.5000000000000000000, 1.000000000000000000 ),
 .UNSPECIFIED. ) ;
#26218=CARTESIAN_POINT ( 'NONE',  ( 8.700000000286459922, -13.45891141627732779, -35.92950628563520610 ) ) ;
#26220=DIRECTION ( 'NONE',  ( -2.764840495839172918E-12, -0.9128796883888953273, 0.4082287037029531107 ) ) ;
#26222=DIRECTION ( 'NONE',  ( 2.764840495839172918E-12, 0.9128796883888953273, -0.4082287037029530552 ) ) ;
#26227=CARTESIAN_POINT ( 'NONE',  ( 8.700000000229927366, -28.07050130669910715, -25.59757157921452020 ) ) ;
#26231=CYLINDRICAL_SURFACE ( 'NONE', #14779, 2.500000000000001776 ) ;
#26243=CARTESIAN_POINT ( 'NONE',  ( 8.350000000651883525, -22.83323352209971091, -39.84673050092360569 ) ) ;
#26249=VERTEX_POINT ( 'NONE', #4212 ) ;
#26250=CARTESIAN_POINT ( 'NONE',  ( 8.700000000229927366, -28.07050130669910715, -25.59757157921452020 ) ) ;
#26257=CARTESIAN_POINT ( 'NONE',  ( 8.700000000277853474, -18.40140086067256320, -36.11849812464715370 ) ) ;
#26261=CARTESIAN_POINT ( 'NONE',  ( 8.000000000291789704, -9.149979919790938609, -35.02638174844400965 ) ) ;
#26274=CARTESIAN_POINT ( 'NONE',  ( 8.700000000248314436, -24.01191590399745479, -28.87649232339336081 ) ) ;
#26286=EDGE_LOOP ( 'NONE', ( #7688, #17810, #9676, #13781, #4852, #19360, #6920, #12649 ) ) ;
#26288=CARTESIAN_POINT ( 'NONE',  ( 4.276011752548591005, -51.11187400310260642, -27.80500476121942199 ) ) ;
#26319=CARTESIAN_POINT ( 'NONE',  ( -7.999999999669004325, -18.23122067930106027, -34.51216076568240965 ) ) ;
#26321=ORIENTED_EDGE ( 'NONE', *, *, #30400, .T. ) ;
#26324=( NAMED_UNIT ( * ) SI_UNIT ( $, .STERADIAN. ) SOLID_ANGLE_UNIT ( ) );
#26330=FACE_BOUND ( 'NONE', #19971, .T. ) ;
#26333=LINE ( 'NONE', #62, #26488 ) ;
#26338=VERTEX_POINT ( 'NONE', #4060 ) ;
#26348=ADVANCED_FACE ( 'NONE', ( #1701 ), #20739, .F. ) ;
#26349=CARTESIAN_POINT ( 'NONE',  ( -8.699999999715885224, -26.99999999997790923, -28.40000000002690683 ) ) ;
#26381=CARTESIAN_POINT ( 'NONE',  ( -7.999999999684150431, -16.34187081459762680, -33.05013248324110720 ) ) ;
#26397=CARTESIAN_POINT ( 'NONE',  ( -8.699999999683917906, -16.84112679184576677, -33.19732076807623145 ) ) ;
#26418=ORIENTED_EDGE ( 'NONE', *, *, #14486, .F. ) ;
#26429=CARTESIAN_POINT ( 'NONE',  ( -7.999999999945165641, -111.9817663798748981, 5.760339591700875950 ) ) ;
#26430=LINE ( 'NONE', #12249, #6217 ) ;
#26435=CARTESIAN_POINT ( 'NONE',  ( -7.999999999654498595, -13.74237167848310115, -36.71272273345665837 ) ) ;
#26459=LINE ( 'NONE', #24102, #14706 ) ;
#26471=CYLINDRICAL_SURFACE ( 'NONE', #21838, 10.00000000000000533 ) ;
#26473=ORIENTED_EDGE ( 'NONE', *, *, #14909, .T. ) ;
#26488=VECTOR ( 'NONE', #7288, 999.9999999999998863 ) ;
#26521=DIRECTION ( 'NONE',  ( -3.924189347185962345E-12, 0.4082287037029530552, 0.9128796883888952163 ) ) ;
#26531=FACE_OUTER_BOUND ( 'NONE', #21042, .T. ) ;
#26546=VECTOR ( 'NONE', #11316, 1000.000000000000000 ) ;
#26550=EDGE_CURVE ( 'NONE', #3906, #26249, #4679, .T. ) ;
#26578=CARTESIAN_POINT ( 'NONE',  ( -7.999999999965972108, -115.9769488450772741, 9.394897729457213131 ) ) ;
#26594=ORIENTED_EDGE ( 'NONE', *, *, #20399, .T. ) ;
#26595=CARTESIAN_POINT ( 'NONE',  ( -7.999999999730326827, -27.47149743197635630, -25.42634137633946878 ) ) ;
#26631=CARTESIAN_POINT ( 'NONE',  ( 8.699999999949548979, -115.5267901941283810, 21.04701626963504069 ) ) ;
#26632=ADVANCED_FACE ( 'NONE', ( #10336 ), #744, .F. ) ;
#26635=FACE_OUTER_BOUND ( 'NONE', #6879, .T. ) ;
#26650=CARTESIAN_POINT ( 'NONE',  ( 8.000000000839454728, -14.48034092994288180, -33.45092210021663703 ) ) ;
#26655=ORIENTED_EDGE ( 'NONE', *, *, #4423, .F. ) ;
#26670=CARTESIAN_POINT ( 'NONE',  ( 8.700000000237631426, -25.41583080867745892, -25.82211739995418753 ) ) ;
#26675=CARTESIAN_POINT ( 'NONE',  ( 8.700000000284820345, -13.66682223737197610, -36.55330428411850363 ) ) ;
#26677=ORIENTED_EDGE ( 'NONE', *, *, #10344, .F. ) ;
#26690=EDGE_CURVE ( 'NONE', #6097, #8184, #13936, .T. ) ;
#26697=FACE_OUTER_BOUND ( 'NONE', #13378, .T. ) ;
#26701=ORIENTED_EDGE ( 'NONE', *, *, #29880, .F. ) ;
#26714=DIRECTION ( 'NONE',  ( -3.924189347185962345E-12, 0.4082287037029530552, 0.9128796883888952163 ) ) ;
#26725=CARTESIAN_POINT ( 'NONE',  ( -7.999999999953479879, -114.0541489762801461, 7.119646953328183869 ) ) ;
#26773=CARTESIAN_POINT ( 'NONE',  ( -7.999999999699952014, -24.42167197178301308, -29.98317312624888231 ) ) ;
#26784=CARTESIAN_POINT ( 'NONE',  ( 8.700000000248671483, -25.22378963206060831, -30.84934466687800025 ) ) ;
#26785=DIRECTION ( 'NONE',  ( 1.667044707805962905E-12, -0.4082287037029530552, -0.9128796883888953273 ) ) ;
#26813=AXIS2_PLACEMENT_3D ( 'NONE', #18529, #13815, #6568 ) ;
#26825=CARTESIAN_POINT ( 'NONE',  ( 8.000000000749292184, -24.01208138067712028, -28.87597782833235627 ) ) ;
#26828=CARTESIAN_POINT ( 'NONE',  ( 8.700000000296723712, -12.54225101349288529, -39.16323275742981025 ) ) ;
#26865=CARTESIAN_POINT ( 'NONE',  ( 8.700000000235451836, -26.13547327700162271, -25.50030203292368114 ) ) ;
#26871=CARTESIAN_POINT ( 'NONE',  ( 8.700000000274457079, -18.36552062635309213, -34.81248186671538036 ) ) ;
#26876=EDGE_LOOP ( 'NONE', ( #6788, #28254, #7999, #19693 ) ) ;
#26882=VECTOR ( 'NONE', #775, 1000.000000000000000 ) ;
#26884=AXIS2_PLACEMENT_3D ( 'NONE', #14708, #16591, #21787 ) ;
#26887=CARTESIAN_POINT ( 'NONE',  ( -7.999999999961045383, -115.3392401410248738, 8.473717002696254497 ) ) ;
#26904=ORIENTED_EDGE ( 'NONE', *, *, #14650, .F. ) ;
#26907=CARTESIAN_POINT ( 'NONE',  ( 8.000000000846746673, -13.86721103371404418, -37.00141305325693963 ) ) ;
#26911=FACE_OUTER_BOUND ( 'NONE', #31063, .T. ) ;
#26926=CARTESIAN_POINT ( 'NONE',  ( -8.699999999726605537, -29.57832802798597527, -26.81682687338189197 ) ) ;
#26934=CARTESIAN_POINT ( 'NONE',  ( 8.000000000488469709, -24.55065533249607412, -26.62378963273996391 ) ) ;
#26938=CARTESIAN_POINT ( 'NONE',  ( -8.699999999691694796, -25.92947359974585098, -31.20249410827203107 ) ) ;
#26939=ORIENTED_EDGE ( 'NONE', *, *, #23388, .F. ) ;
#26947=CARTESIAN_POINT ( 'NONE',  ( -8.000000000050450311, -115.5267901941129907, 21.04701626955636939 ) ) ;
#26967=CARTESIAN_POINT ( 'NONE',  ( -8.699999999675917195, -17.42919676355489855, -33.49161196806937824 ) ) ;
#27028=ORIENTED_EDGE ( 'NONE', *, *, #30294, .T. ) ;
#27035=CARTESIAN_POINT ( 'NONE',  ( 8.700000000270996736, -18.23122067931645773, -34.51216076560373125 ) ) ;
#27039=CARTESIAN_POINT ( 'NONE',  ( -8.699999999694114194, -28.22468611108677194, -31.13863906519358693 ) ) ;
#27052=ORIENTED_EDGE ( 'NONE', *, *, #8216, .F. ) ;
#27055=VERTEX_POINT ( 'NONE', #20352 ) ;
#27073=DIRECTION ( 'NONE',  ( 2.764840495839172918E-12, 0.9128796883888953273, -0.4082287037029531107 ) ) ;
#27082=AXIS2_PLACEMENT_3D ( 'NONE', #27602, #10617, #19911 ) ;
#27086=CARTESIAN_POINT ( 'NONE',  ( 7.000000000277405654, -5.572998883592096497, -27.02754848641193419 ) ) ;
#27099=ORIENTED_EDGE ( 'NONE', *, *, #20120, .F. ) ;
#27105=EDGE_LOOP ( 'NONE', ( #28915, #3850, #22258, #8742 ) ) ;
#27115=LINE ( 'NONE', #17052, #7670 ) ;
#27129=ORIENTED_EDGE ( 'NONE', *, *, #1198, .F. ) ;
#27133=ORIENTED_EDGE ( 'NONE', *, *, #20399, .F. ) ;
#27181=DIRECTION ( 'NONE',  ( 2.416122857340496113E-12, -0.9341647027306024809, -0.3568421334038978099 ) ) ;
#27186=EDGE_CURVE ( 'NONE', #6080, #19159, #29714, .T. ) ;
#27192=EDGE_CURVE ( 'NONE', #19512, #6463, #17593, .T. ) ;
#27198=ORIENTED_EDGE ( 'NONE', *, *, #23830, .F. ) ;
#27201=CARTESIAN_POINT ( 'NONE',  ( -8.699999999675029017, -13.90762120762749809, -34.05293844846480056 ) ) ;
#27209=CARTESIAN_POINT ( 'NONE',  ( 1.057488903014505443E-10, -103.0613381315276484, 16.56805218638653798 ) ) ;
#27235=LINE ( 'NONE', #5675, #24889 ) ;
#27247=EDGE_CURVE ( 'NONE', #30387, #368, #21916, .T. ) ;
#27248=CARTESIAN_POINT ( 'NONE',  ( -7.999999999659703320, -18.25871770053183596, -36.49215491283803914 ) ) ;
#27254=CARTESIAN_POINT ( 'NONE',  ( -7.665314379701609226, -5.675505773878507298, -27.25677405838692735 ) ) ;
#27270=VECTOR ( 'NONE', #8836, 999.9999999999998863 ) ;
#27315=EDGE_CURVE ( 'NONE', #14873, #9577, #17575, .T. ) ;
#27322=ADVANCED_FACE ( 'NONE', ( #10046 ), #19489, .F. ) ;
#27328=CARTESIAN_POINT ( 'NONE',  ( -7.000000000054375171, -115.1185614904109542, 21.95989595794997129 ) ) ;
#27331=CARTESIAN_POINT ( 'NONE',  ( 8.700000000280979862, -17.99038303693934893, -37.01276636704596967 ) ) ;
#27348=AXIS2_PLACEMENT_3D ( 'NONE', #18003, #1512, #6532 ) ;
#27391=CARTESIAN_POINT ( 'NONE',  ( 7.998464191499309983, -115.5020148795422728, 21.10241874685433672 ) ) ;
#27392=ORIENTED_EDGE ( 'NONE', *, *, #4249, .F. ) ;
#27398=ORIENTED_EDGE ( 'NONE', *, *, #22431, .F. ) ;
#27429=EDGE_CURVE ( 'NONE', #15836, #12111, #12398, .T. ) ;
#27435=CARTESIAN_POINT ( 'NONE',  ( -8.000000000030556890, -116.5561065465021784, 18.74526241810166027 ) ) ;
#27444=ORIENTED_EDGE ( 'NONE', *, *, #6739, .F. ) ;
#27457=B_SPLINE_CURVE_WITH_KNOTS ( 'NONE', 3,
 ( #2609, #10161, #268, #24169, #29501, #7486 ),
 .UNSPECIFIED., .F., .F.,
 ( 4, 2, 4 ),
 ( 0.000000000000000000, 0.5000000000000000000, 1.000000000000000000 ),
 .UNSPECIFIED. ) ;
#27478=CARTESIAN_POINT ( 'NONE',  ( -8.000000000477658801, -25.77531388886969310, -25.66136093485691916 ) ) ;
#27499=CARTESIAN_POINT ( 'NONE',  ( -8.699999999674142614, -13.61360970150653316, -34.64062719139432289 ) ) ;
#27518=EDGE_CURVE ( 'NONE', #30584, #4237, #13652, .T. ) ;
#27529=CARTESIAN_POINT ( 'NONE',  ( -8.699999999668968087, -13.49637763710977900, -34.94770709601201020 ) ) ;
#27534=EDGE_LOOP ( 'NONE', ( #18109, #11384, #18578, #8221 ) ) ;
#27535=B_SPLINE_CURVE_WITH_KNOTS ( 'NONE', 4,
 ( #25519, #3956, #23161, #1602, #11192 ),
 .UNSPECIFIED., .F., .F.,
 ( 5, 5 ),
 ( -0.9817477042469999748, 0.9817477042469999748 ),
 .UNSPECIFIED. ) ;
#27537=CARTESIAN_POINT ( 'NONE',  ( 8.699999999502342263, -25.77531388888509056, -25.66136093477824431 ) ) ;
#27573=CARTESIAN_POINT ( 'NONE',  ( -8.699999999655181782, -13.66682223737418944, -36.55330428419230060 ) ) ;
#27590=CARTESIAN_POINT ( 'NONE',  ( -8.699999999628365899, -17.59709758660007139, -40.94395633085227360 ) ) ;
#27598=VERTEX_POINT ( 'NONE', #4516 ) ;
#27602=CARTESIAN_POINT ( 'NONE',  ( 5.797918471924832673, -115.0360660102050048, 22.14437208032004989 ) ) ;
#27610=CYLINDRICAL_SURFACE ( 'NONE', #19811, 3.000000000000002220 ) ;
#27641=CARTESIAN_POINT ( 'NONE',  ( -8.699999999715885224, -26.99999999997790923, -28.40000000002690683 ) ) ;
#27650=LINE ( 'NONE', #2016, #9287 ) ;
#27707=CARTESIAN_POINT ( 'NONE',  ( -7.291979204152452709, -5.587697461206379224, -27.06041739756416931 ) ) ;
#27723=ADVANCED_FACE ( 'NONE', ( #16311 ), #4358, .F. ) ;
#27730=VERTEX_POINT ( 'NONE', #29185 ) ;
#27758=DIRECTION ( 'NONE',  ( -2.764840495839172918E-12, -0.9128796883888953273, 0.4082287037029531107 ) ) ;
#27776=CYLINDRICAL_SURFACE ( 'NONE', #16209, 3.000000000000002220 ) ;
#27785=ORIENTED_EDGE ( 'NONE', *, *, #1198, .T. ) ;
#27790=ADVANCED_FACE ( 'NONE', ( #26531 ), #2770, .F. ) ;
#27806=AXIS2_PLACEMENT_3D ( 'NONE', #21804, #17453, #22503 ) ;
#27816=EDGE_LOOP ( 'NONE', ( #6265, #5132, #21748, #18806, #9910 ) ) ;
#27821=EDGE_CURVE ( 'NONE', #24850, #15988, #27457, .T. ) ;
#27825=FILL_AREA_STYLE ('',( #23440 ) ) ;
#27844=VECTOR ( 'NONE', #2430, 1000.000000000000000 ) ;
#27857=CARTESIAN_POINT ( 'NONE',  ( -8.699999998944143442, -13.61360970150653316, -34.64062719139432289 ) ) ;
#27863=VERTEX_POINT ( 'NONE', #21971 ) ;
#27877=EDGE_LOOP ( 'NONE', ( #30935, #29658, #11763, #24082 ) ) ;
#27897=EDGE_LOOP ( 'NONE', ( #13939, #15741, #12337, #17488 ) ) ;
#27926=LINE ( 'NONE', #20852, #21729 ) ;
#27929=CARTESIAN_POINT ( 'NONE',  ( -8.699999999685100960, -16.20661859040315989, -33.02459860127090252 ) ) ;
#27943=CARTESIAN_POINT ( 'NONE',  ( 7.707106781468556100, -5.692566302608600637, -27.29492475672613594 ) ) ;
#27952=DIRECTION ( 'NONE',  ( 0.000000000000000000, -0.9128796883888953273, 0.4082287037029528332 ) ) ;
#27963=DIRECTION ( 'NONE',  ( -1.000000000000000000, 9.219999999999999084E-13, -4.710999999999999616E-12 ) ) ;
#27982=EDGE_LOOP ( 'NONE', ( #9348, #29985, #14223, #9126 ) ) ;
#27984=DIRECTION ( 'NONE',  ( -2.764840495839172918E-12, -0.9128796883888953273, 0.4082287037029530552 ) ) ;
#28008=EDGE_LOOP ( 'NONE', ( #13727, #23739, #29402, #14491 ) ) ;
#28021=CARTESIAN_POINT ( 'NONE',  ( 8.700000000276082446, -16.84110654130126150, -33.19737377701691372 ) ) ;
#28039=CARTESIAN_POINT ( 'NONE',  ( -7.999999999691694619, -25.92947359974649046, -31.20249410826873415 ) ) ;
#28054=EDGE_CURVE ( 'NONE', #24719, #1905, #28699, .T. ) ;
#28056=ORIENTED_EDGE ( 'NONE', *, *, #19079, .F. ) ;
#28087=CARTESIAN_POINT ( 'NONE',  ( -8.700000000014243895, -117.3672015282731280, 16.33620429947759334 ) ) ;
#28091=AXIS2_PLACEMENT_3D ( 'NONE', #21497, #22117, #29339 ) ;
#28103=ORIENTED_EDGE ( 'NONE', *, *, #18072, .T. ) ;
#28107=AXIS2_PLACEMENT_3D ( 'NONE', #12780, #13077, #22079 ) ;
#28119=DIRECTION ( 'NONE',  ( -1.000000000000000000, 5.687697913155423197E-16, -6.771501495041734442E-12 ) ) ;
#28127=AXIS2_PLACEMENT_3D ( 'NONE', #27209, #25603, #27952 ) ;
#28139=ORIENTED_EDGE ( 'NONE', *, *, #12770, .F. ) ;
#28146=CARTESIAN_POINT ( 'NONE',  ( 8.000000000285856672, -13.61361098174325868, -34.64062768040190576 ) ) ;
#28185=VERTEX_POINT ( 'NONE', #29466 ) ;
#28191=CARTESIAN_POINT ( 'NONE',  ( -7.505215711015759794, -115.1705934733524543, 21.84354220833749949 ) ) ;
#28198=VERTEX_POINT ( 'NONE', #22398 ) ;
#28209=ORIENTED_EDGE ( 'NONE', *, *, #2152, .F. ) ;
#28214=CARTESIAN_POINT ( 'NONE',  ( -8.699999999629611125, -16.25267700569241569, -40.75987951459011782 ) ) ;
#28219=CARTESIAN_POINT ( 'NONE',  ( -8.699999999715885224, -26.99999999997790923, -28.40000000002690683 ) ) ;
#28254=ORIENTED_EDGE ( 'NONE', *, *, #6721, .F. ) ;
#28256=VECTOR ( 'NONE', #29305, 1000.000000000000000 ) ;
#28263=CARTESIAN_POINT ( 'NONE',  ( -8.699999999662093586, -15.94902145834643115, -35.53273252493492862 ) ) ;
#28306=EDGE_CURVE ( 'NONE', #16100, #11991, #13990, .T. ) ;
#28312=CARTESIAN_POINT ( 'NONE',  ( 8.700000000289357160, -13.80041476817676127, -36.85204346332353254 ) ) ;
#28318=VECTOR ( 'NONE', #14286, 1000.000000000000000 ) ;
#28323=ORIENTED_EDGE ( 'NONE', *, *, #12082, .T. ) ;
#28345=AXIS2_PLACEMENT_3D ( 'NONE', #24632, #5583, #14889 ) ;
#28349=CARTESIAN_POINT ( 'NONE',  ( -7.000000000054375171, -115.1185614904109542, 21.95989595794997129 ) ) ;
#28366=ORIENTED_EDGE ( 'NONE', *, *, #23117, .T. ) ;
#28369=EDGE_LOOP ( 'NONE', ( #28417, #29244, #19899, #21438 ) ) ;
#28371=SURFACE_STYLE_USAGE ( .BOTH. , #4460 ) ;
#28372=VECTOR ( 'NONE', #29269, 1000.000000000000000 ) ;
#28378=CARTESIAN_POINT ( 'NONE',  ( -8.699999999654229654, -13.99314194387733323, -37.12415143712361498 ) ) ;
#28381=DIRECTION ( 'NONE',  ( 1.000000000000000000, -9.224647189900200933E-13, 4.710284450064084831E-12 ) ) ;
#28417=ORIENTED_EDGE ( 'NONE', *, *, #12082, .F. ) ;
#28426=EDGE_CURVE ( 'NONE', #27863, #368, #188, .T. ) ;
#28453=B_SPLINE_CURVE_WITH_KNOTS ( 'NONE', 3,
 ( #2459, #14725, #12505, #26218, #12052, #26675 ),
 .UNSPECIFIED., .F., .F.,
 ( 4, 2, 4 ),
 ( 0.000000000000000000, 0.5000000000000000000, 1.000000000000000000 ),
 .UNSPECIFIED. ) ;
#28460=EDGE_LOOP ( 'NONE', ( #31006, #27052, #5560, #3369 ) ) ;
#28472=CARTESIAN_POINT ( 'NONE',  ( 8.700000000234771491, -29.98808444042839838, -27.92350772035144857 ) ) ;
#28476=CYLINDRICAL_SURFACE ( 'NONE', #11456, 3.000000000000002220 ) ;
#28487=ADVANCED_FACE ( 'NONE', ( #8478 ), #22513, .T. ) ;
#28511=ORIENTED_EDGE ( 'NONE', *, *, #6621, .F. ) ;
#28517=EDGE_LOOP ( 'NONE', ( #1789, #824, #597, #19476 ) ) ;
#28519=DIRECTION ( 'NONE',  ( 1.000000000000000000, -1.843431230200657634E-12, 2.650498504950726461E-12 ) ) ;
#28541=ADVANCED_FACE ( 'NONE', ( #17914 ), #10863, .F. ) ;
#28548=EDGE_CURVE ( 'NONE', #2785, #3623, #25970, .T. ) ;
#28554=CARTESIAN_POINT ( 'NONE',  ( 2.660567502109009752E-10, -9.320059656530233383, -25.35190844155029311 ) ) ;
#28604=EDGE_CURVE ( 'NONE', #10911, #13888, #20330, .T. ) ;
#28611=CARTESIAN_POINT ( 'NONE',  ( 8.000000000250498289, -24.42231254078294000, -29.98460556443784952 ) ) ;
#28613=CARTESIAN_POINT ( 'NONE',  ( -8.699999999633741155, -14.31588153610736036, -40.15003283749538099 ) ) ;
#28686=B_SPLINE_CURVE_WITH_KNOTS ( 'NONE', 5,
 ( #835, #29614, #8048, #989, #20480, #16074, #18107, #29925, #10723 ),
 .UNSPECIFIED., .F., .F.,
 ( 6, 3, 6 ),
 ( 0.000000000000000000, 1.646696145469999983, 2.782752055940000080 ),
 .UNSPECIFIED. ) ;
#28688=CARTESIAN_POINT ( 'NONE',  ( -7.999999999695856623, -18.27877680370596636, -30.94409471158115110 ) ) ;
#28695=DIRECTION ( 'NONE',  ( 2.764840495839172918E-12, 0.9128796883888953273, -0.4082287037029531107 ) ) ;
#28696=CARTESIAN_POINT ( 'NONE',  ( -8.699999999711218734, -30.00985298778766008, -28.70958934910558469 ) ) ;
#28699=LINE ( 'NONE', #18632, #5230 ) ;
#28701=CARTESIAN_POINT ( 'NONE',  ( 8.000000000285856672, -13.61361098174325868, -34.64062768040190576 ) ) ;
#28711=VERTEX_POINT ( 'NONE', #4015 ) ;
#28713=VERTEX_POINT ( 'NONE', #20861 ) ;
#28740=CYLINDRICAL_SURFACE ( 'NONE', #5271, 3.000000000000002220 ) ;
#28788=AXIS2_PLACEMENT_3D ( 'NONE', #14323, #16657, #23923 ) ;
#28811=EDGE_CURVE ( 'NONE', #17179, #24995, #18749, .T. ) ;
#28821=ORIENTED_EDGE ( 'NONE', *, *, #19672, .T. ) ;
#28831=VECTOR ( 'NONE', #30667, 999.9999999999998863 ) ;
#28840=CARTESIAN_POINT ( 'NONE',  ( -8.699999999884559188, -60.75400889059604737, -3.446705952705766407 ) ) ;
#28856=VECTOR ( 'NONE', #30731, 1000.000000000000000 ) ;
#28862=ORIENTED_EDGE ( 'NONE', *, *, #16369, .F. ) ;
#28866=CARTESIAN_POINT ( 'NONE',  ( 8.000000000287716517, -16.96959321760095563, -37.81493174583665251 ) ) ;
#28874=B_SPLINE_CURVE_WITH_KNOTS ( 'NONE', 3,
 ( #12917, #22527, #8178, #972, #26773, #20158 ),
 .UNSPECIFIED., .F., .F.,
 ( 4, 2, 4 ),
 ( 0.000000000000000000, 0.5000000000000000000, 1.000000000000000000 ),
 .UNSPECIFIED. ) ;
#28884=FACE_OUTER_BOUND ( 'NONE', #25504, .T. ) ;
#28890=CARTESIAN_POINT ( 'NONE',  ( -7.999999999786640892, -67.40749995144636841, -17.04319545400304392 ) ) ;
#28915=ORIENTED_EDGE ( 'NONE', *, *, #13726, .F. ) ;
#28929=CARTESIAN_POINT ( 'NONE',  ( -8.699999999696727215, -25.22421763345087342, -30.84970730147981754 ) ) ;
#28990=DIRECTION ( 'NONE',  ( 0.000000000000000000, -0.9128796883888949942, 0.4082287037029534438 ) ) ;
#28999=AXIS2_PLACEMENT_3D ( 'NONE', #14413, #5109, #3055 ) ;
#29017=ORIENTED_EDGE ( 'NONE', *, *, #107, .F. ) ;
#29028=CARTESIAN_POINT ( 'NONE',  ( 8.700000000241349341, -24.55027189127212850, -26.62408091262140530 ) ) ;
#29032=CARTESIAN_POINT ( 'NONE',  ( -7.999999999643747195, -11.71436167353443736, -38.59800651357252121 ) ) ;
#29037=ORIENTED_EDGE ( 'NONE', *, *, #10251, .T. ) ;
#29043=CARTESIAN_POINT ( 'NONE',  ( -8.699999999725333666, -24.55029269852046170, -26.62421763350704040 ) ) ;
#29053=DIRECTION ( 'NONE',  ( -3.134067079931429195E-12, -0.3568421334038983650, 0.9341647027306021478 ) ) ;
#29054=CARTESIAN_POINT ( 'NONE',  ( 7.195957064175671825, -115.1234601580806611, 21.94894157346885066 ) ) ;
#29059=ORIENTED_EDGE ( 'NONE', *, *, #10079, .F. ) ;
#29074=ORIENTED_EDGE ( 'NONE', *, *, #24442, .F. ) ;
#29087=CARTESIAN_POINT ( 'NONE',  ( -7.999999999982724042, -116.6191538659648188, 10.70265178694466002 ) ) ;
#29181=CARTESIAN_POINT ( 'NONE',  ( -7.999999999684021645, -16.70556587905094759, -33.14831771973513241 ) ) ;
#29185=CARTESIAN_POINT ( 'NONE',  ( -8.000000000457589522, -24.26136093481186862, -29.62468611113247263 ) ) ;
#29195=CARTESIAN_POINT ( 'NONE',  ( -7.999999999674821005, -13.66746466538290328, -34.50691966471094929 ) ) ;
#29196=EDGE_CURVE ( 'NONE', #11537, #2785, #2280, .T. ) ;
#29203=DIRECTION ( 'NONE',  ( 1.000000000000000000, 0.000000000000000000, 0.000000000000000000 ) ) ;
#29212=EDGE_CURVE ( 'NONE', #22033, #30387, #20658, .T. ) ;
#29213=( NAMED_UNIT ( * ) PLANE_ANGLE_UNIT ( ) SI_UNIT ( $, .RADIAN. ) );
#29222=VECTOR ( 'NONE', #829, 999.9999999999998863 ) ;
#29226=AXIS2_PLACEMENT_3D ( 'NONE', #28219, #16260, #4314 ) ;
#29244=ORIENTED_EDGE ( 'NONE', *, *, #4048, .F. ) ;
#29254=CARTESIAN_POINT ( 'NONE',  ( 8.000000000479330353, -14.59835909869570081, -37.69297980903808565 ) ) ;
#29269=DIRECTION ( 'NONE',  ( -1.000000000000000000, 5.687697999151106851E-16, -6.771501495036750356E-12 ) ) ;
#29288=ORIENTED_EDGE ( 'NONE', *, *, #17652, .F. ) ;
#29304=CARTESIAN_POINT ( 'NONE',  ( 8.000000000279957391, -18.28443193505134445, -36.42483736938841332 ) ) ;
#29305=DIRECTION ( 'NONE',  ( 1.000000000000000000, -1.841917067661885521E-12, 2.653884470265303553E-12 ) ) ;
#29328=CARTESIAN_POINT ( 'NONE',  ( -8.000000000026910030, -116.9355502247062617, 17.89675170932962089 ) ) ;
#29329=ORIENTED_EDGE ( 'NONE', *, *, #21960, .F. ) ;
#29337=CARTESIAN_POINT ( 'NONE',  ( -7.999999999682374074, -15.09104283142151282, -33.18208307865850060 ) ) ;
#29339=DIRECTION ( 'NONE',  ( 2.764802276011834743E-12, 0.9128796883888953273, -0.4082287037029531662 ) ) ;
#29340=ORIENTED_EDGE ( 'NONE', *, *, #7644, .F. ) ;
#29367=AXIS2_PLACEMENT_3D ( 'NONE', #20448, #6125, #15719 ) ;
#29380=STYLED_ITEM ( 'NONE', ( #25554 ), #17044 ) ;
#29397=EDGE_CURVE ( 'NONE', #15988, #23469, #14317, .T. ) ;
#29402=ORIENTED_EDGE ( 'NONE', *, *, #16435, .T. ) ;
#29429=CARTESIAN_POINT ( 'NONE',  ( -7.973786364210958766, -115.4211104591501993, 21.28333694629189665 ) ) ;
#29435=ADVANCED_FACE ( 'NONE', ( #11172 ), #3938, .F. ) ;
#29442=CARTESIAN_POINT ( 'NONE',  ( 7.707106507606773960, -115.2381290211091738, 21.69251943803729787 ) ) ;
#29466=CARTESIAN_POINT ( 'NONE',  ( 8.000000000248304488, -25.92947504235655032, -31.20249033167290165 ) ) ;
#29471=CARTESIAN_POINT ( 'NONE',  ( -7.999999999703424791, -29.80249410822368006, -29.47052640025566816 ) ) ;
#29483=CARTESIAN_POINT ( 'NONE',  ( -7.999999999991574740, -117.2096321409668462, 12.46567123851033010 ) ) ;
#29489=EDGE_CURVE ( 'NONE', #17596, #19970, #26430, .T. ) ;
#29491=CARTESIAN_POINT ( 'NONE',  ( -7.999999999661212335, -10.00744863972343168, -36.67931076521506384 ) ) ;
#29493=UNCERTAINTY_MEASURE_WITH_UNIT (LENGTH_MEASURE( 1.000000000000000082E-05 ), #11540, 'distance_accuracy_value', 'NONE');
#29496=EDGE_CURVE ( 'NONE', #28711, #7680, #16913, .T. ) ;
#29501=CARTESIAN_POINT ( 'NONE',  ( 8.700000000291131741, -15.36262080770071670, -37.98492059649628771 ) ) ;
#29509=DIRECTION ( 'NONE',  ( -6.181427515845962162E-12, 0.4082287037029531107, 0.9128796883888953273 ) ) ;
#29511=CARTESIAN_POINT ( 'NONE',  ( -7.999999999680079021, -14.41853751394117111, -33.53780267086614231 ) ) ;
#29532=CARTESIAN_POINT ( 'NONE',  ( 8.350000000354834029, -111.9817663810069774, 5.760339591729700004 ) ) ;
#29561=ORIENTED_EDGE ( 'NONE', *, *, #29196, .F. ) ;
#29600=DIRECTION ( 'NONE',  ( -2.764840495839172918E-12, -0.9128796883888953273, 0.4082287037029530552 ) ) ;
#29614=CARTESIAN_POINT ( 'NONE',  ( -7.999999999656092875, -13.57196071827068096, -36.34117526632622486 ) ) ;
#29644=EDGE_LOOP ( 'NONE', ( #7119, #25288, #25074, #22218, #16614, #19349, #19868, #12923 ) ) ;
#29645=PLANE ( 'NONE',  #12958 ) ;
#29648=EDGE_CURVE ( 'NONE', #23341, #21601, #13747, .T. ) ;
#29654=VERTEX_POINT ( 'NONE', #27039 ) ;
#29658=ORIENTED_EDGE ( 'NONE', *, *, #20299, .T. ) ;
#29673=ADVANCED_FACE ( 'NONE', ( #10984 ), #3113, .F. ) ;
#29694=VERTEX_POINT ( 'NONE', #29855 ) ;
#29714=LINE ( 'NONE', #24687, #11261 ) ;
#29717=ORIENTED_EDGE ( 'NONE', *, *, #12770, .T. ) ;
#29737=CARTESIAN_POINT ( 'NONE',  ( -8.699999998977590465, -24.26136093481122558, -29.62468611113576955 ) ) ;
#29745=CARTESIAN_POINT ( 'NONE',  ( -8.349999999680450813, -115.5267901938268977, 21.04701627019373333 ) ) ;
#29801=B_SPLINE_CURVE_WITH_KNOTS ( 'NONE', 5,
 ( #5591, #22130, #29195, #21980, #24798, #24643, #22282, #29511, #19771, #739, #10629, #436 ),
 .UNSPECIFIED., .F., .F.,
 ( 6, 3, 3, 6 ),
 ( 2.782752055940000080, 3.293393369179999919, 4.940089939870000002, 5.565010778459999585 ),
 .UNSPECIFIED. ) ;
#29810=DIRECTION ( 'NONE',  ( 2.764802276011834339E-12, 0.9128796883888953273, -0.4082287037029531107 ) ) ;
#29818=AXIS2_PLACEMENT_3D ( 'NONE', #7952, #24956, #22604 ) ;
#29835=FACE_OUTER_BOUND ( 'NONE', #18613, .T. ) ;
#29840=CARTESIAN_POINT ( 'NONE',  ( -8.699999999718343702, -24.19750589173278499, -27.32947359979484858 ) ) ;
#29855=CARTESIAN_POINT ( 'NONE',  ( 8.700000000278096834, -14.92844969908683517, -33.25053330388887218 ) ) ;
#29879=CARTESIAN_POINT ( 'NONE',  ( 8.000000000842893755, -13.46643344106513318, -36.10519551497034030 ) ) ;
#29880=EDGE_CURVE ( 'NONE', #6080, #10105, #5987, .T. ) ;
#29895=DIRECTION ( 'NONE',  ( -1.000000000000000000, 5.687697999151106851E-16, -6.771501495036750356E-12 ) ) ;
#29923=FACE_OUTER_BOUND ( 'NONE', #26167, .T. ) ;
#29925=CARTESIAN_POINT ( 'NONE',  ( -7.999999999673383044, -13.55640290378411095, -34.79039326168094703 ) ) ;
#29938=CYLINDRICAL_SURFACE ( 'NONE', #13814, 2.500000000000000888 ) ;
#29950=DIRECTION ( 'NONE',  ( -2.764840495839172918E-12, -0.9128796883888953273, 0.4082287037029530552 ) ) ;
#29957=CARTESIAN_POINT ( 'NONE',  ( -4.276011752261355880, -9.320059656537083015, -25.35190844156560885 ) ) ;
#29958=DIRECTION ( 'NONE',  ( -1.000000000000000000, 5.687697958343395332E-16, -6.771501495045879231E-12 ) ) ;
#29984=CARTESIAN_POINT ( 'NONE',  ( -8.699999999731023337, -27.70368077816327101, -25.45737431350073265 ) ) ;
#29985=ORIENTED_EDGE ( 'NONE', *, *, #6805, .F. ) ;
#30001=CARTESIAN_POINT ( 'NONE',  ( -7.999999999718343524, -24.19750589173343869, -27.32947359979155166 ) ) ;
#30013=B_SPLINE_CURVE_WITH_KNOTS ( 'NONE', 3,
 ( #1331, #8386, #8549, #1646, #20519, #6359 ),
 .UNSPECIFIED., .F., .F.,
 ( 4, 2, 4 ),
 ( 0.000000000000000000, 0.4999999999999997780, 1.000000000000000000 ),
 .UNSPECIFIED. ) ;
#30019=EDGE_LOOP ( 'NONE', ( #5407, #25316, #18941, #20424 ) ) ;
#30022=ORIENTED_EDGE ( 'NONE', *, *, #5775, .T. ) ;
#30048=AXIS2_PLACEMENT_3D ( 'NONE', #14213, #26171, #9799 ) ;
#30050=CARTESIAN_POINT ( 'NONE',  ( -8.699999999666752970, -13.44080163377184256, -35.27486921256096508 ) ) ;
#30058=EDGE_LOOP ( 'NONE', ( #1978, #24048, #3711, #10159 ) ) ;
#30068=ADVANCED_FACE ( 'NONE', ( #9155 ), #19075, .F. ) ;
#30080=CARTESIAN_POINT ( 'NONE',  ( -7.097978819962594166, -5.572998883415808180, -27.02754848611320071 ) ) ;
#30101=VERTEX_POINT ( 'NONE', #4452 ) ;
#30108=ORIENTED_EDGE ( 'NONE', *, *, #3047, .F. ) ;
#30111=EDGE_LOOP ( 'NONE', ( #26939, #19096, #11266, #4726 ) ) ;
#30131=CARTESIAN_POINT ( 'NONE',  ( 7.999999999977091214, -107.4273096626279482, 14.66297538114749344 ) ) ;
#30137=EDGE_CURVE ( 'NONE', #90, #29694, #10126, .T. ) ;
#30177=VERTEX_POINT ( 'NONE', #23964 ) ;
#30179=ORIENTED_EDGE ( 'NONE', *, *, #6074, .T. ) ;
#30180=EDGE_CURVE ( 'NONE', #22622, #23040, #4595, .T. ) ;
#30192=CARTESIAN_POINT ( 'NONE',  ( -8.699999999985950083, -116.8589940772574920, 11.34037319969351643 ) ) ;
#30193=CARTESIAN_POINT ( 'NONE',  ( 7.707106507606773960, -115.2381290211091738, 21.69251943803729787 ) ) ;
#30202=CARTESIAN_POINT ( 'NONE',  ( -8.000000000319866800, -28.58317312641834462, -30.97832802812172659 ) ) ;
#30209=ORIENTED_EDGE ( 'NONE', *, *, #30982, .F. ) ;
#30210=EDGE_CURVE ( 'NONE', #15161, #17525, #20973, .T. ) ;
#30227=CARTESIAN_POINT ( 'NONE',  ( -8.699999999000075590, -28.07052640020997458, -25.59750589178178259 ) ) ;
#30245=AXIS2_PLACEMENT_3D ( 'NONE', #26027, #18774, #28381 ) ;
#30256=EDGE_CURVE ( 'NONE', #16606, #30101, #360, .T. ) ;
#30268=B_SPLINE_CURVE_WITH_KNOTS ( 'NONE', 3,
 ( #25771, #3730, #1541, #11446, #10976, #30001 ),
 .UNSPECIFIED., .F., .F.,
 ( 4, 2, 4 ),
 ( 0.000000000000000000, 0.5000000000000000000, 1.000000000000000000 ),
 .UNSPECIFIED. ) ;
#30269=ORIENTED_EDGE ( 'NONE', *, *, #30256, .F. ) ;
#30293=CARTESIAN_POINT ( 'NONE',  ( 8.700000000277906764, -15.94902145836247342, -35.53273252485295330 ) ) ;
#30294=EDGE_CURVE ( 'NONE', #3623, #16606, #1729, .T. ) ;
#30303=DIRECTION ( 'NONE',  ( -1.000000000000000000, 5.687698019339887572E-16, -6.771501495046482653E-12 ) ) ;
#30322=ORIENTED_EDGE ( 'NONE', *, *, #6805, .T. ) ;
#30347=EDGE_LOOP ( 'NONE', ( #16398, #1561, #9557, #11215 ) ) ;
#30354=FACE_OUTER_BOUND ( 'NONE', #1116, .T. ) ;
#30374=VECTOR ( 'NONE', #13376, 1000.000000000000000 ) ;
#30378=CARTESIAN_POINT ( 'NONE',  ( 8.700000000289733748, -15.05693637256081097, -37.86809127166881694 ) ) ;
#30387=VERTEX_POINT ( 'NONE', #12138 ) ;
#30400=EDGE_CURVE ( 'NONE', #1828, #15932, #20848, .T. ) ;
#30414=CARTESIAN_POINT ( 'NONE',  ( 7.000000000115440102, -60.75400889061052112, -3.446705952631804681 ) ) ;
#30430=LINE ( 'NONE', #13899, #4795 ) ;
#30433=EDGE_LOOP ( 'NONE', ( #8175, #19202, #10725, #6653 ) ) ;
#30437=EDGE_CURVE ( 'NONE', #6463, #16921, #10559, .T. ) ;
#30463=CARTESIAN_POINT ( 'NONE',  ( 8.350000000381330167, -5.981227587133004064, -27.94042817442931792 ) ) ;
#30468=ORIENTED_EDGE ( 'NONE', *, *, #6531, .T. ) ;
#30470=EDGE_CURVE ( 'NONE', #3623, #18002, #13062, .T. ) ;
#30485=UNCERTAINTY_MEASURE_WITH_UNIT (LENGTH_MEASURE( 1.000000000000000082E-05 ), #24196, 'distance_accuracy_value', 'NONE');
#30491=CARTESIAN_POINT ( 'NONE',  ( -8.699999999718343702, -24.19750589173278499, -27.32947359979484858 ) ) ;
#30520=CARTESIAN_POINT ( 'NONE',  ( 8.699999999551790708, -9.149979919791583427, -35.02638174844071983 ) ) ;
#30540=CARTESIAN_POINT ( 'NONE',  ( 7.000000000115440102, -60.75400889061052112, -3.446705952631804681 ) ) ;
#30543=ORIENTED_EDGE ( 'NONE', *, *, #28604, .T. ) ;
#30550=LINE ( 'NONE', #30227, #7525 ) ;
#30576=ORIENTED_EDGE ( 'NONE', *, *, #10797, .T. ) ;
#30579=CARTESIAN_POINT ( 'NONE',  ( 1.814857447021396585E-10, -110.9401521129946389, -1.050525799519145487 ) ) ;
#30584=VERTEX_POINT ( 'NONE', #16096 ) ;
#30610=CARTESIAN_POINT ( 'NONE',  ( -8.699999999684971286, -15.55237326750320825, -33.04280034228838048 ) ) ;
#30630=CIRCLE ( 'NONE', #3471, 4.276011752367109509 ) ;
#30643=CARTESIAN_POINT ( 'NONE',  ( 8.000000000277404766, -5.572998883593017538, -27.02754848640722329 ) ) ;
#30647=CYLINDRICAL_SURFACE ( 'NONE', #9138, 1.000000000000001110 ) ;
#30661=ORIENTED_EDGE ( 'NONE', *, *, #1903, .F. ) ;
#30665=CARTESIAN_POINT ( 'NONE',  ( -8.699999999730072986, -28.07050130677435362, -25.59757157925566773 ) ) ;
#30667=DIRECTION ( 'NONE',  ( -2.764840495839172918E-12, -0.9128796883888953273, 0.4082287037029531107 ) ) ;
#30676=ORIENTED_EDGE ( 'NONE', *, *, #8704, .F. ) ;
#30682=CARTESIAN_POINT ( 'NONE',  ( -7.999999999628196967, -15.17858304667434233, -40.45432020020274422 ) ) ;
#30685=CARTESIAN_POINT ( 'NONE',  ( 8.700000000284820345, -13.66682223737197610, -36.55330428411850363 ) ) ;
#30695=ORIENTED_EDGE ( 'NONE', *, *, #14909, .F. ) ;
#30705=B_SPLINE_CURVE_WITH_KNOTS ( 'NONE', 3,
 ( #9166, #8858, #23195, #23041, #6504, #18768 ),
 .UNSPECIFIED., .F., .F.,
 ( 4, 2, 4 ),
 ( 0.000000000000000000, 0.5000000000000000000, 1.000000000000000000 ),
 .UNSPECIFIED. ) ;
#30731=DIRECTION ( 'NONE',  ( 1.000000000000000000, -1.843431230200084908E-12, 2.650498504963248473E-12 ) ) ;
#30739=EDGE_CURVE ( 'NONE', #11537, #19543, #21286, .T. ) ;
#30761=VERTEX_POINT ( 'NONE', #7276 ) ;
#30768=DIRECTION ( 'NONE',  ( 1.000000000000000000, -1.843431230200084908E-12, 2.650498504963248473E-12 ) ) ;
#30788=CARTESIAN_POINT ( 'NONE',  ( 8.700000000244243026, -28.90935745820462088, -30.74712106076765394 ) ) ;
#30796=ADVANCED_FACE ( 'NONE', ( #5066 ), #26471, .T. ) ;
#30810=VERTEX_POINT ( 'NONE', #52 ) ;
#30816=CARTESIAN_POINT ( 'NONE',  ( -8.000000000054376059, -115.1185614904100447, 21.95989595794526039 ) ) ;
#30838=DIRECTION ( 'NONE',  ( -2.249415931299125355E-12, 0.9431856258987900699, 0.3322662713817151059 ) ) ;
#30844=CARTESIAN_POINT ( 'NONE',  ( 8.700000000281329804, -5.981227587278358016, -27.94042817480098506 ) ) ;
#30869=AXIS2_PLACEMENT_3D ( 'NONE', #24836, #5937, #10664 ) ;
#30912=ORIENTED_EDGE ( 'NONE', *, *, #23117, .F. ) ;
#30925=B_SPLINE_CURVE_WITH_KNOTS ( 'NONE', 3,
 ( #13639, #23244, #30788, #23872, #9213, #6552 ),
 .UNSPECIFIED., .F., .F.,
 ( 4, 2, 4 ),
 ( 0.000000000000000000, 0.5000000000000000000, 1.000000000000000000 ),
 .UNSPECIFIED. ) ;
#30935=ORIENTED_EDGE ( 'NONE', *, *, #3884, .F. ) ;
#30936=DIRECTION ( 'NONE',  ( 6.181422929335961825E-12, -0.4082287037029531107, -0.9128796883888953273 ) ) ;
#30947=FACE_OUTER_BOUND ( 'NONE', #30111, .T. ) ;
#30951=CARTESIAN_POINT ( 'NONE',  ( 8.700000000231774777, -28.77591908717043268, -25.95027189104346732 ) ) ;
#30967=EDGE_LOOP ( 'NONE', ( #20943, #10270, #1943, #23778, #16668 ) ) ;
#30970=EDGE_CURVE ( 'NONE', #29654, #11652, #8446, .T. ) ;
#30972=CARTESIAN_POINT ( 'NONE',  ( -8.699999999635686265, -13.70503196073122965, -39.86243280111477105 ) ) ;
#30982=EDGE_CURVE ( 'NONE', #3651, #14873, #3550, .T. ) ;
#31006=ORIENTED_EDGE ( 'NONE', *, *, #7815, .F. ) ;
#31008=VERTEX_POINT ( 'NONE', #20306 ) ;
#31011=CARTESIAN_POINT ( 'NONE',  ( -7.999999999628359504, -14.95611408987656965, -40.37595097054163773 ) ) ;
#31018=B_SPLINE_CURVE_WITH_KNOTS ( 'NONE', 3,
 ( #12908, #26926, #5362, #17617, #17766, #14967 ),
 .UNSPECIFIED., .F., .F.,
 ( 4, 2, 4 ),
 ( 0.000000000000000000, 0.5000000000000000000, 1.000000000000000000 ),
 .UNSPECIFIED. ) ;
#31053=AXIS2_PLACEMENT_3D ( 'NONE', #7955, #3390, #15362 ) ;
#31063=EDGE_LOOP ( 'NONE', ( #20908, #1705, #18177, #28103, #203 ) ) ;
#31064=CARTESIAN_POINT ( 'NONE',  ( 8.000000000742927497, -28.90964379103893123, -30.74680062208867071 ) ) ;
#31095=VECTOR ( 'NONE', #469, 999.9999999999998863 ) ;
#31117=CARTESIAN_POINT ( 'NONE',  ( -8.699999999668209583, -9.149979920083866958, -35.02638174926116221 ) ) ;
ENDSEC;
END-ISO-10303-21;
